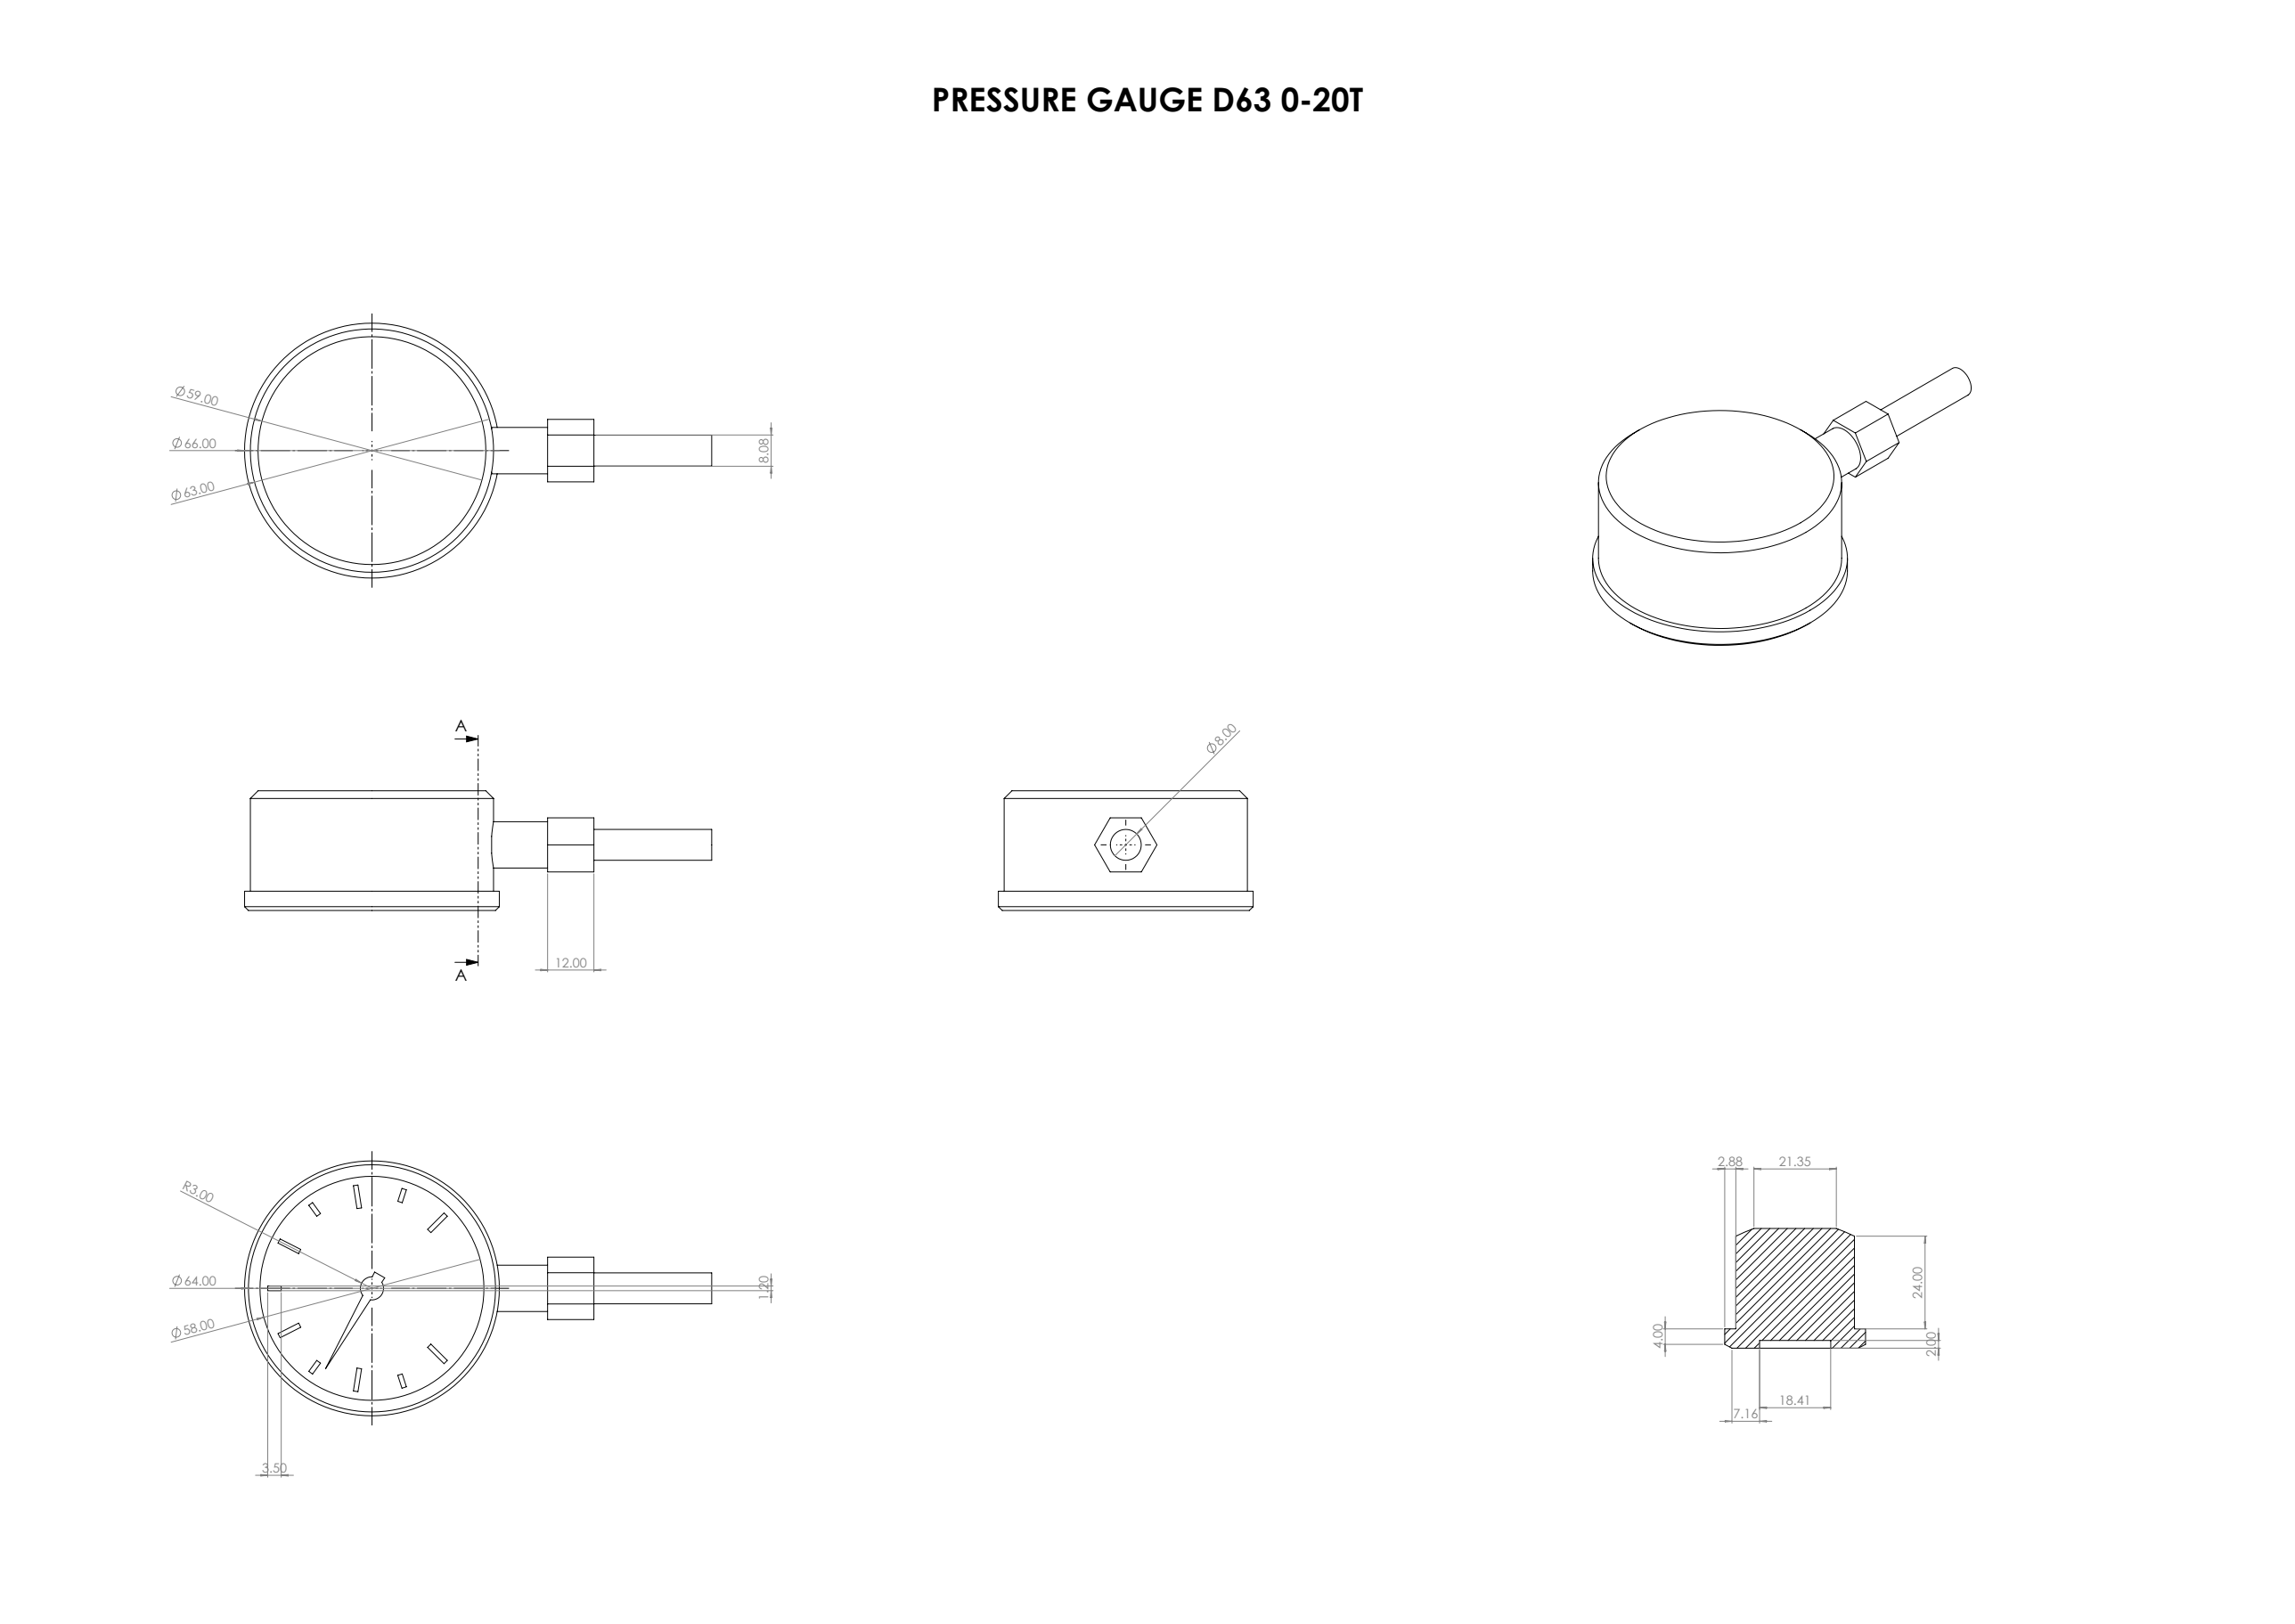
ISO-10303-21;
HEADER;
/* Generated by software containing ST-Developer
 * from STEP Tools, Inc. (www.steptools.com) 
 */

FILE_DESCRIPTION(
/* description */ (''),
/* implementation_level */ '2;1');

FILE_NAME(
/* name */ '13_Pressure_Gauge_D63_0-20T.step',
/* time_stamp */ '2026-10-20T10:03:03-07:00',
/* author */ (''),
/* organization */ (''),
/* preprocessor_version */ 'ST-DEVELOPER v20.2',
/* originating_system */ 'Autodesk Translation Framework v15.15.0.0',
/* authorisation */ '');

FILE_SCHEMA (('AUTOMOTIVE_DESIGN { 1 0 10303 214 3 1 1 }'));
ENDSEC;

DATA;
#10=MECHANICAL_DESIGN_GEOMETRIC_PRESENTATION_REPRESENTATION('',(#531,#532),#71492);
#389=SHAPE_REPRESENTATION_RELATIONSHIP('SRR','None',#71610,#408);
#408=ADVANCED_BREP_SHAPE_REPRESENTATION('',(#427),#71480);
#427=MANIFOLD_SOLID_BREP('Gauge',#28466);
#531=STYLED_ITEM('',(#71901),#27845);
#532=STYLED_ITEM('',(#71901),#427);
#878=B_SPLINE_CURVE_WITH_KNOTS('',3,(#48749,#48750,#48751,#48752,#48753,
#48754,#48755,#48756,#48757,#48758,#48759,#48760,#48761,#48762,#48763,#48764,
#48765,#48766),.UNSPECIFIED.,.F.,.F.,(4,2,2,2,2,2,2,2,4),(0.214479017187888,
0.226613658149299,0.453227316298599,0.679830564793567,0.906433813288534,
1.1330370617835,1.35964031027847,1.58625396842777,1.59838860938918),
 .UNSPECIFIED.);
#879=B_SPLINE_CURVE_WITH_KNOTS('',3,(#48768,#48769,#48770,#48771,#48772,
#48773,#48774,#48775,#48776,#48777,#48778,#48779,#48780,#48781,#48782,#48783,
#48784,#48785),.UNSPECIFIED.,.F.,.F.,(4,2,2,2,2,2,2,2,4),(2.02734664376496,
2.03948128472637,2.26609494287567,2.49269819137064,2.7193014398656,2.94590468836057,
3.17250793685554,3.39912159500484,3.41125623596625),.UNSPECIFIED.);
#1661=CYLINDRICAL_SURFACE('',#29879,0.4);
#1662=CYLINDRICAL_SURFACE('',#29897,0.6);
#1663=CYLINDRICAL_SURFACE('',#29898,0.300000000000001);
#1664=CYLINDRICAL_SURFACE('',#29904,0.300000000000001);
#1665=CYLINDRICAL_SURFACE('',#29967,2.9);
#1666=CYLINDRICAL_SURFACE('',#29973,3.15);
#1667=CYLINDRICAL_SURFACE('',#29977,3.3);
#1931=FACE_BOUND('',#5501,.T.);
#1932=FACE_BOUND('',#5509,.T.);
#1933=FACE_BOUND('',#5577,.T.);
#1934=FACE_BOUND('',#5578,.T.);
#1935=FACE_BOUND('',#5579,.T.);
#1936=FACE_BOUND('',#5580,.T.);
#1937=FACE_BOUND('',#5581,.T.);
#1938=FACE_BOUND('',#5582,.T.);
#1939=FACE_BOUND('',#5583,.T.);
#1940=FACE_BOUND('',#5584,.T.);
#1941=FACE_BOUND('',#5585,.T.);
#1942=FACE_BOUND('',#5586,.T.);
#1943=FACE_BOUND('',#5587,.T.);
#1944=FACE_BOUND('',#5588,.T.);
#1945=FACE_BOUND('',#5593,.T.);
#1946=FACE_BOUND('',#5595,.T.);
#1947=FACE_BOUND('',#5599,.T.);
#2447=CIRCLE('',#29880,0.4);
#2448=CIRCLE('',#29881,0.4);
#2449=CIRCLE('',#29884,0.6);
#2450=CIRCLE('',#29893,0.6);
#2451=CIRCLE('',#29895,0.6);
#2452=CIRCLE('',#29896,0.6);
#2453=CIRCLE('',#29899,0.300000000000001);
#2454=CIRCLE('',#29900,0.300000000000001);
#2455=CIRCLE('',#29905,0.300000000000001);
#2456=CIRCLE('',#29906,0.300000000000001);
#2457=CIRCLE('',#29966,2.9);
#2458=CIRCLE('',#29968,2.9);
#2459=CIRCLE('',#29970,2.95);
#2460=CIRCLE('',#29972,3.15);
#2461=CIRCLE('',#29974,3.15);
#2462=CIRCLE('',#29976,3.3);
#2463=CIRCLE('',#29978,3.3);
#2464=CIRCLE('',#29980,3.2);
#2859=CONICAL_SURFACE('',#29971,3.05,0.785398163397449);
#2860=CONICAL_SURFACE('',#29979,3.25,0.785398163397447);
#3861=FACE_OUTER_BOUND('',#5498,.T.);
#3862=FACE_OUTER_BOUND('',#5499,.T.);
#3863=FACE_OUTER_BOUND('',#5500,.T.);
#3864=FACE_OUTER_BOUND('',#5502,.T.);
#3865=FACE_OUTER_BOUND('',#5503,.T.);
#3866=FACE_OUTER_BOUND('',#5504,.T.);
#3867=FACE_OUTER_BOUND('',#5505,.T.);
#3868=FACE_OUTER_BOUND('',#5506,.T.);
#3869=FACE_OUTER_BOUND('',#5507,.T.);
#3870=FACE_OUTER_BOUND('',#5508,.T.);
#3871=FACE_OUTER_BOUND('',#5510,.T.);
#3872=FACE_OUTER_BOUND('',#5511,.T.);
#3873=FACE_OUTER_BOUND('',#5512,.T.);
#3874=FACE_OUTER_BOUND('',#5513,.T.);
#3875=FACE_OUTER_BOUND('',#5514,.T.);
#3876=FACE_OUTER_BOUND('',#5515,.T.);
#3877=FACE_OUTER_BOUND('',#5516,.T.);
#3878=FACE_OUTER_BOUND('',#5517,.T.);
#3879=FACE_OUTER_BOUND('',#5518,.T.);
#3880=FACE_OUTER_BOUND('',#5519,.T.);
#3881=FACE_OUTER_BOUND('',#5520,.T.);
#3882=FACE_OUTER_BOUND('',#5521,.T.);
#3883=FACE_OUTER_BOUND('',#5522,.T.);
#3884=FACE_OUTER_BOUND('',#5523,.T.);
#3885=FACE_OUTER_BOUND('',#5524,.T.);
#3886=FACE_OUTER_BOUND('',#5525,.T.);
#3887=FACE_OUTER_BOUND('',#5526,.T.);
#3888=FACE_OUTER_BOUND('',#5527,.T.);
#3889=FACE_OUTER_BOUND('',#5528,.T.);
#3890=FACE_OUTER_BOUND('',#5529,.T.);
#3891=FACE_OUTER_BOUND('',#5530,.T.);
#3892=FACE_OUTER_BOUND('',#5531,.T.);
#3893=FACE_OUTER_BOUND('',#5532,.T.);
#3894=FACE_OUTER_BOUND('',#5533,.T.);
#3895=FACE_OUTER_BOUND('',#5534,.T.);
#3896=FACE_OUTER_BOUND('',#5535,.T.);
#3897=FACE_OUTER_BOUND('',#5536,.T.);
#3898=FACE_OUTER_BOUND('',#5537,.T.);
#3899=FACE_OUTER_BOUND('',#5538,.T.);
#3900=FACE_OUTER_BOUND('',#5539,.T.);
#3901=FACE_OUTER_BOUND('',#5540,.T.);
#3902=FACE_OUTER_BOUND('',#5541,.T.);
#3903=FACE_OUTER_BOUND('',#5542,.T.);
#3904=FACE_OUTER_BOUND('',#5543,.T.);
#3905=FACE_OUTER_BOUND('',#5544,.T.);
#3906=FACE_OUTER_BOUND('',#5545,.T.);
#3907=FACE_OUTER_BOUND('',#5546,.T.);
#3908=FACE_OUTER_BOUND('',#5547,.T.);
#3909=FACE_OUTER_BOUND('',#5548,.T.);
#3910=FACE_OUTER_BOUND('',#5549,.T.);
#3911=FACE_OUTER_BOUND('',#5550,.T.);
#3912=FACE_OUTER_BOUND('',#5551,.T.);
#3913=FACE_OUTER_BOUND('',#5552,.T.);
#3914=FACE_OUTER_BOUND('',#5553,.T.);
#3915=FACE_OUTER_BOUND('',#5554,.T.);
#3916=FACE_OUTER_BOUND('',#5555,.T.);
#3917=FACE_OUTER_BOUND('',#5556,.T.);
#3918=FACE_OUTER_BOUND('',#5557,.T.);
#3919=FACE_OUTER_BOUND('',#5558,.T.);
#3920=FACE_OUTER_BOUND('',#5559,.T.);
#3921=FACE_OUTER_BOUND('',#5560,.T.);
#3922=FACE_OUTER_BOUND('',#5561,.T.);
#3923=FACE_OUTER_BOUND('',#5562,.T.);
#3924=FACE_OUTER_BOUND('',#5563,.T.);
#3925=FACE_OUTER_BOUND('',#5564,.T.);
#3926=FACE_OUTER_BOUND('',#5565,.T.);
#3927=FACE_OUTER_BOUND('',#5566,.T.);
#3928=FACE_OUTER_BOUND('',#5567,.T.);
#3929=FACE_OUTER_BOUND('',#5568,.T.);
#3930=FACE_OUTER_BOUND('',#5569,.T.);
#3931=FACE_OUTER_BOUND('',#5570,.T.);
#3932=FACE_OUTER_BOUND('',#5571,.T.);
#3933=FACE_OUTER_BOUND('',#5572,.T.);
#3934=FACE_OUTER_BOUND('',#5573,.T.);
#3935=FACE_OUTER_BOUND('',#5574,.T.);
#3936=FACE_OUTER_BOUND('',#5575,.T.);
#3937=FACE_OUTER_BOUND('',#5576,.T.);
#3938=FACE_OUTER_BOUND('',#5589,.T.);
#3939=FACE_OUTER_BOUND('',#5590,.T.);
#3940=FACE_OUTER_BOUND('',#5591,.T.);
#3941=FACE_OUTER_BOUND('',#5592,.T.);
#3942=FACE_OUTER_BOUND('',#5594,.T.);
#3943=FACE_OUTER_BOUND('',#5596,.T.);
#3944=FACE_OUTER_BOUND('',#5597,.T.);
#3945=FACE_OUTER_BOUND('',#5598,.T.);
#5498=EDGE_LOOP('',(#22583,#22584,#22585,#22586));
#5499=EDGE_LOOP('',(#22587));
#5500=EDGE_LOOP('',(#22588,#22589,#22590,#22591,#22592,#22593));
#5501=EDGE_LOOP('',(#22594));
#5502=EDGE_LOOP('',(#22595,#22596,#22597,#22598));
#5503=EDGE_LOOP('',(#22599,#22600,#22601,#22602));
#5504=EDGE_LOOP('',(#22603,#22604,#22605,#22606));
#5505=EDGE_LOOP('',(#22607,#22608,#22609,#22610));
#5506=EDGE_LOOP('',(#22611,#22612,#22613,#22614));
#5507=EDGE_LOOP('',(#22615,#22616,#22617,#22618));
#5508=EDGE_LOOP('',(#22619,#22620,#22621,#22622,#22623,#22624));
#5509=EDGE_LOOP('',(#22625));
#5510=EDGE_LOOP('',(#22626,#22627));
#5511=EDGE_LOOP('',(#22628,#22629,#22630));
#5512=EDGE_LOOP('',(#22631,#22632,#22633,#22634,#22635,#22636,#22637,#22638));
#5513=EDGE_LOOP('',(#22639,#22640,#22641,#22642));
#5514=EDGE_LOOP('',(#22643,#22644,#22645,#22646));
#5515=EDGE_LOOP('',(#22647,#22648,#22649,#22650));
#5516=EDGE_LOOP('',(#22651,#22652,#22653,#22654));
#5517=EDGE_LOOP('',(#22655,#22656,#22657,#22658));
#5518=EDGE_LOOP('',(#22659,#22660,#22661,#22662));
#5519=EDGE_LOOP('',(#22663,#22664,#22665,#22666));
#5520=EDGE_LOOP('',(#22667,#22668,#22669,#22670,#22671,#22672,#22673));
#5521=EDGE_LOOP('',(#22674,#22675,#22676,#22677));
#5522=EDGE_LOOP('',(#22678,#22679,#22680,#22681));
#5523=EDGE_LOOP('',(#22682,#22683,#22684,#22685));
#5524=EDGE_LOOP('',(#22686,#22687,#22688,#22689));
#5525=EDGE_LOOP('',(#22690,#22691,#22692,#22693));
#5526=EDGE_LOOP('',(#22694,#22695,#22696,#22697));
#5527=EDGE_LOOP('',(#22698,#22699,#22700,#22701));
#5528=EDGE_LOOP('',(#22702,#22703,#22704,#22705));
#5529=EDGE_LOOP('',(#22706,#22707,#22708,#22709));
#5530=EDGE_LOOP('',(#22710,#22711,#22712,#22713));
#5531=EDGE_LOOP('',(#22714,#22715,#22716,#22717));
#5532=EDGE_LOOP('',(#22718,#22719,#22720,#22721));
#5533=EDGE_LOOP('',(#22722,#22723,#22724,#22725));
#5534=EDGE_LOOP('',(#22726,#22727,#22728,#22729));
#5535=EDGE_LOOP('',(#22730,#22731,#22732,#22733));
#5536=EDGE_LOOP('',(#22734,#22735,#22736,#22737));
#5537=EDGE_LOOP('',(#22738,#22739,#22740,#22741));
#5538=EDGE_LOOP('',(#22742,#22743,#22744,#22745));
#5539=EDGE_LOOP('',(#22746,#22747,#22748,#22749));
#5540=EDGE_LOOP('',(#22750,#22751,#22752,#22753));
#5541=EDGE_LOOP('',(#22754,#22755,#22756,#22757));
#5542=EDGE_LOOP('',(#22758,#22759,#22760,#22761));
#5543=EDGE_LOOP('',(#22762,#22763,#22764,#22765));
#5544=EDGE_LOOP('',(#22766,#22767,#22768,#22769));
#5545=EDGE_LOOP('',(#22770,#22771,#22772,#22773));
#5546=EDGE_LOOP('',(#22774,#22775,#22776,#22777));
#5547=EDGE_LOOP('',(#22778,#22779,#22780,#22781));
#5548=EDGE_LOOP('',(#22782,#22783,#22784,#22785));
#5549=EDGE_LOOP('',(#22786,#22787,#22788,#22789));
#5550=EDGE_LOOP('',(#22790,#22791,#22792,#22793));
#5551=EDGE_LOOP('',(#22794,#22795,#22796,#22797));
#5552=EDGE_LOOP('',(#22798,#22799,#22800,#22801));
#5553=EDGE_LOOP('',(#22802,#22803,#22804,#22805));
#5554=EDGE_LOOP('',(#22806,#22807,#22808,#22809));
#5555=EDGE_LOOP('',(#22810,#22811,#22812,#22813));
#5556=EDGE_LOOP('',(#22814,#22815,#22816,#22817));
#5557=EDGE_LOOP('',(#22818,#22819,#22820,#22821));
#5558=EDGE_LOOP('',(#22822,#22823,#22824,#22825));
#5559=EDGE_LOOP('',(#22826,#22827,#22828,#22829));
#5560=EDGE_LOOP('',(#22830,#22831,#22832,#22833));
#5561=EDGE_LOOP('',(#22834,#22835,#22836,#22837));
#5562=EDGE_LOOP('',(#22838,#22839,#22840,#22841));
#5563=EDGE_LOOP('',(#22842,#22843,#22844,#22845));
#5564=EDGE_LOOP('',(#22846,#22847,#22848,#22849));
#5565=EDGE_LOOP('',(#22850,#22851,#22852,#22853));
#5566=EDGE_LOOP('',(#22854,#22855,#22856,#22857));
#5567=EDGE_LOOP('',(#22858,#22859,#22860,#22861));
#5568=EDGE_LOOP('',(#22862,#22863,#22864,#22865));
#5569=EDGE_LOOP('',(#22866,#22867,#22868,#22869));
#5570=EDGE_LOOP('',(#22870,#22871,#22872,#22873));
#5571=EDGE_LOOP('',(#22874,#22875,#22876,#22877));
#5572=EDGE_LOOP('',(#22878,#22879,#22880,#22881));
#5573=EDGE_LOOP('',(#22882,#22883,#22884,#22885));
#5574=EDGE_LOOP('',(#22886,#22887,#22888,#22889));
#5575=EDGE_LOOP('',(#22890,#22891,#22892,#22893));
#5576=EDGE_LOOP('',(#22894));
#5577=EDGE_LOOP('',(#22895,#22896,#22897,#22898));
#5578=EDGE_LOOP('',(#22899,#22900,#22901,#22902));
#5579=EDGE_LOOP('',(#22903,#22904,#22905,#22906));
#5580=EDGE_LOOP('',(#22907,#22908,#22909,#22910));
#5581=EDGE_LOOP('',(#22911,#22912,#22913,#22914));
#5582=EDGE_LOOP('',(#22915,#22916,#22917,#22918));
#5583=EDGE_LOOP('',(#22919,#22920,#22921,#22922));
#5584=EDGE_LOOP('',(#22923,#22924,#22925,#22926));
#5585=EDGE_LOOP('',(#22927,#22928,#22929,#22930));
#5586=EDGE_LOOP('',(#22931,#22932,#22933,#22934));
#5587=EDGE_LOOP('',(#22935,#22936,#22937,#22938));
#5588=EDGE_LOOP('',(#22939,#22940,#22941,#22942,#22943,#22944,#22945));
#5589=EDGE_LOOP('',(#22946,#22947,#22948,#22949));
#5590=EDGE_LOOP('',(#22950));
#5591=EDGE_LOOP('',(#22951,#22952,#22953,#22954));
#5592=EDGE_LOOP('',(#22955,#22956,#22957,#22958));
#5593=EDGE_LOOP('',(#22959,#22960,#22961,#22962));
#5594=EDGE_LOOP('',(#22963));
#5595=EDGE_LOOP('',(#22964));
#5596=EDGE_LOOP('',(#22965,#22966,#22967,#22968));
#5597=EDGE_LOOP('',(#22969,#22970,#22971,#22972));
#5598=EDGE_LOOP('',(#22973));
#5599=EDGE_LOOP('',(#22974));
#7821=LINE('',#48693,#10309);
#7822=LINE('',#48699,#10310);
#7823=LINE('',#48701,#10311);
#7824=LINE('',#48703,#10312);
#7825=LINE('',#48705,#10313);
#7826=LINE('',#48707,#10314);
#7827=LINE('',#48708,#10315);
#7828=LINE('',#48714,#10316);
#7829=LINE('',#48715,#10317);
#7830=LINE('',#48716,#10318);
#7831=LINE('',#48719,#10319);
#7832=LINE('',#48720,#10320);
#7833=LINE('',#48723,#10321);
#7834=LINE('',#48724,#10322);
#7835=LINE('',#48727,#10323);
#7836=LINE('',#48728,#10324);
#7837=LINE('',#48731,#10325);
#7838=LINE('',#48732,#10326);
#7839=LINE('',#48734,#10327);
#7840=LINE('',#48739,#10328);
#7841=LINE('',#48744,#10329);
#7842=LINE('',#48767,#10330);
#7843=LINE('',#48791,#10331);
#7844=LINE('',#48794,#10332);
#7845=LINE('',#48797,#10333);
#7846=LINE('',#48799,#10334);
#7847=LINE('',#48800,#10335);
#7848=LINE('',#48803,#10336);
#7849=LINE('',#48805,#10337);
#7850=LINE('',#48806,#10338);
#7851=LINE('',#48809,#10339);
#7852=LINE('',#48811,#10340);
#7853=LINE('',#48812,#10341);
#7854=LINE('',#48818,#10342);
#7855=LINE('',#48821,#10343);
#7856=LINE('',#48823,#10344);
#7857=LINE('',#48824,#10345);
#7858=LINE('',#48826,#10346);
#7859=LINE('',#48827,#10347);
#7860=LINE('',#48832,#10348);
#7861=LINE('',#48834,#10349);
#7862=LINE('',#48836,#10350);
#7863=LINE('',#48837,#10351);
#7864=LINE('',#48840,#10352);
#7865=LINE('',#48842,#10353);
#7866=LINE('',#48843,#10354);
#7867=LINE('',#48846,#10355);
#7868=LINE('',#48848,#10356);
#7869=LINE('',#48849,#10357);
#7870=LINE('',#48851,#10358);
#7871=LINE('',#48852,#10359);
#7872=LINE('',#48857,#10360);
#7873=LINE('',#48859,#10361);
#7874=LINE('',#48861,#10362);
#7875=LINE('',#48862,#10363);
#7876=LINE('',#48865,#10364);
#7877=LINE('',#48867,#10365);
#7878=LINE('',#48868,#10366);
#7879=LINE('',#48871,#10367);
#7880=LINE('',#48873,#10368);
#7881=LINE('',#48874,#10369);
#7882=LINE('',#48876,#10370);
#7883=LINE('',#48877,#10371);
#7884=LINE('',#48882,#10372);
#7885=LINE('',#48884,#10373);
#7886=LINE('',#48886,#10374);
#7887=LINE('',#48887,#10375);
#7888=LINE('',#48890,#10376);
#7889=LINE('',#48892,#10377);
#7890=LINE('',#48893,#10378);
#7891=LINE('',#48896,#10379);
#7892=LINE('',#48898,#10380);
#7893=LINE('',#48899,#10381);
#7894=LINE('',#48901,#10382);
#7895=LINE('',#48902,#10383);
#7896=LINE('',#48907,#10384);
#7897=LINE('',#48909,#10385);
#7898=LINE('',#48911,#10386);
#7899=LINE('',#48912,#10387);
#7900=LINE('',#48915,#10388);
#7901=LINE('',#48917,#10389);
#7902=LINE('',#48918,#10390);
#7903=LINE('',#48921,#10391);
#7904=LINE('',#48923,#10392);
#7905=LINE('',#48924,#10393);
#7906=LINE('',#48926,#10394);
#7907=LINE('',#48927,#10395);
#7908=LINE('',#48932,#10396);
#7909=LINE('',#48934,#10397);
#7910=LINE('',#48936,#10398);
#7911=LINE('',#48937,#10399);
#7912=LINE('',#48940,#10400);
#7913=LINE('',#48942,#10401);
#7914=LINE('',#48943,#10402);
#7915=LINE('',#48946,#10403);
#7916=LINE('',#48948,#10404);
#7917=LINE('',#48949,#10405);
#7918=LINE('',#48951,#10406);
#7919=LINE('',#48952,#10407);
#7920=LINE('',#48957,#10408);
#7921=LINE('',#48959,#10409);
#7922=LINE('',#48961,#10410);
#7923=LINE('',#48962,#10411);
#7924=LINE('',#48965,#10412);
#7925=LINE('',#48967,#10413);
#7926=LINE('',#48968,#10414);
#7927=LINE('',#48971,#10415);
#7928=LINE('',#48973,#10416);
#7929=LINE('',#48974,#10417);
#7930=LINE('',#48976,#10418);
#7931=LINE('',#48977,#10419);
#7932=LINE('',#48982,#10420);
#7933=LINE('',#48984,#10421);
#7934=LINE('',#48986,#10422);
#7935=LINE('',#48987,#10423);
#7936=LINE('',#48990,#10424);
#7937=LINE('',#48992,#10425);
#7938=LINE('',#48993,#10426);
#7939=LINE('',#48996,#10427);
#7940=LINE('',#48998,#10428);
#7941=LINE('',#48999,#10429);
#7942=LINE('',#49001,#10430);
#7943=LINE('',#49002,#10431);
#7944=LINE('',#49007,#10432);
#7945=LINE('',#49009,#10433);
#7946=LINE('',#49011,#10434);
#7947=LINE('',#49012,#10435);
#7948=LINE('',#49015,#10436);
#7949=LINE('',#49017,#10437);
#7950=LINE('',#49018,#10438);
#7951=LINE('',#49021,#10439);
#7952=LINE('',#49023,#10440);
#7953=LINE('',#49024,#10441);
#7954=LINE('',#49026,#10442);
#7955=LINE('',#49027,#10443);
#7956=LINE('',#49032,#10444);
#7957=LINE('',#49034,#10445);
#7958=LINE('',#49036,#10446);
#7959=LINE('',#49037,#10447);
#7960=LINE('',#49040,#10448);
#7961=LINE('',#49042,#10449);
#7962=LINE('',#49043,#10450);
#7963=LINE('',#49046,#10451);
#7964=LINE('',#49048,#10452);
#7965=LINE('',#49049,#10453);
#7966=LINE('',#49051,#10454);
#7967=LINE('',#49052,#10455);
#7968=LINE('',#49057,#10456);
#7969=LINE('',#49059,#10457);
#7970=LINE('',#49061,#10458);
#7971=LINE('',#49062,#10459);
#7972=LINE('',#49065,#10460);
#7973=LINE('',#49067,#10461);
#7974=LINE('',#49068,#10462);
#7975=LINE('',#49071,#10463);
#7976=LINE('',#49073,#10464);
#7977=LINE('',#49074,#10465);
#7978=LINE('',#49076,#10466);
#7979=LINE('',#49077,#10467);
#7980=LINE('',#49082,#10468);
#7981=LINE('',#49084,#10469);
#7982=LINE('',#49086,#10470);
#7983=LINE('',#49087,#10471);
#7984=LINE('',#49090,#10472);
#7985=LINE('',#49092,#10473);
#7986=LINE('',#49093,#10474);
#7987=LINE('',#49096,#10475);
#7988=LINE('',#49098,#10476);
#7989=LINE('',#49099,#10477);
#7990=LINE('',#49101,#10478);
#7991=LINE('',#49102,#10479);
#7992=LINE('',#49109,#10480);
#7993=LINE('',#49117,#10481);
#7994=LINE('',#49121,#10482);
#7995=LINE('',#49128,#10483);
#7996=LINE('',#49132,#10484);
#10309=VECTOR('',#34760,0.4);
#10310=VECTOR('',#34767,1.);
#10311=VECTOR('',#34768,1.);
#10312=VECTOR('',#34769,1.);
#10313=VECTOR('',#34770,1.);
#10314=VECTOR('',#34771,1.);
#10315=VECTOR('',#34772,1.);
#10316=VECTOR('',#34777,1.);
#10317=VECTOR('',#34778,1.);
#10318=VECTOR('',#34779,1.);
#10319=VECTOR('',#34782,1.);
#10320=VECTOR('',#34783,1.);
#10321=VECTOR('',#34786,1.);
#10322=VECTOR('',#34787,1.);
#10323=VECTOR('',#34790,1.);
#10324=VECTOR('',#34791,1.);
#10325=VECTOR('',#34794,1.);
#10326=VECTOR('',#34795,1.);
#10327=VECTOR('',#34798,1.);
#10328=VECTOR('',#34803,1.);
#10329=VECTOR('',#34808,1.);
#10330=VECTOR('',#34815,0.6);
#10331=VECTOR('',#34820,1.);
#10332=VECTOR('',#34823,1.);
#10333=VECTOR('',#34826,1.);
#10334=VECTOR('',#34827,1.);
#10335=VECTOR('',#34828,1.);
#10336=VECTOR('',#34831,1.);
#10337=VECTOR('',#34832,1.);
#10338=VECTOR('',#34833,1.);
#10339=VECTOR('',#34836,1.);
#10340=VECTOR('',#34837,1.);
#10341=VECTOR('',#34838,1.);
#10342=VECTOR('',#34845,1.);
#10343=VECTOR('',#34848,1.);
#10344=VECTOR('',#34849,1.);
#10345=VECTOR('',#34850,1.);
#10346=VECTOR('',#34853,1.);
#10347=VECTOR('',#34854,1.);
#10348=VECTOR('',#34859,1.);
#10349=VECTOR('',#34860,1.);
#10350=VECTOR('',#34861,1.);
#10351=VECTOR('',#34862,1.);
#10352=VECTOR('',#34865,1.);
#10353=VECTOR('',#34866,1.);
#10354=VECTOR('',#34867,1.);
#10355=VECTOR('',#34870,1.);
#10356=VECTOR('',#34871,1.);
#10357=VECTOR('',#34872,1.);
#10358=VECTOR('',#34875,1.);
#10359=VECTOR('',#34876,1.);
#10360=VECTOR('',#34881,1.);
#10361=VECTOR('',#34882,1.);
#10362=VECTOR('',#34883,1.);
#10363=VECTOR('',#34884,1.);
#10364=VECTOR('',#34887,1.);
#10365=VECTOR('',#34888,1.);
#10366=VECTOR('',#34889,1.);
#10367=VECTOR('',#34892,1.);
#10368=VECTOR('',#34893,1.);
#10369=VECTOR('',#34894,1.);
#10370=VECTOR('',#34897,1.);
#10371=VECTOR('',#34898,1.);
#10372=VECTOR('',#34903,1.);
#10373=VECTOR('',#34904,1.);
#10374=VECTOR('',#34905,1.);
#10375=VECTOR('',#34906,1.);
#10376=VECTOR('',#34909,1.);
#10377=VECTOR('',#34910,1.);
#10378=VECTOR('',#34911,1.);
#10379=VECTOR('',#34914,1.);
#10380=VECTOR('',#34915,1.);
#10381=VECTOR('',#34916,1.);
#10382=VECTOR('',#34919,1.);
#10383=VECTOR('',#34920,1.);
#10384=VECTOR('',#34925,1.);
#10385=VECTOR('',#34926,1.);
#10386=VECTOR('',#34927,1.);
#10387=VECTOR('',#34928,1.);
#10388=VECTOR('',#34931,1.);
#10389=VECTOR('',#34932,1.);
#10390=VECTOR('',#34933,1.);
#10391=VECTOR('',#34936,1.);
#10392=VECTOR('',#34937,1.);
#10393=VECTOR('',#34938,1.);
#10394=VECTOR('',#34941,1.);
#10395=VECTOR('',#34942,1.);
#10396=VECTOR('',#34947,1.);
#10397=VECTOR('',#34948,1.);
#10398=VECTOR('',#34949,1.);
#10399=VECTOR('',#34950,1.);
#10400=VECTOR('',#34953,1.);
#10401=VECTOR('',#34954,1.);
#10402=VECTOR('',#34955,1.);
#10403=VECTOR('',#34958,1.);
#10404=VECTOR('',#34959,1.);
#10405=VECTOR('',#34960,1.);
#10406=VECTOR('',#34963,1.);
#10407=VECTOR('',#34964,1.);
#10408=VECTOR('',#34969,1.);
#10409=VECTOR('',#34970,1.);
#10410=VECTOR('',#34971,1.);
#10411=VECTOR('',#34972,1.);
#10412=VECTOR('',#34975,1.);
#10413=VECTOR('',#34976,1.);
#10414=VECTOR('',#34977,1.);
#10415=VECTOR('',#34980,1.);
#10416=VECTOR('',#34981,1.);
#10417=VECTOR('',#34982,1.);
#10418=VECTOR('',#34985,1.);
#10419=VECTOR('',#34986,1.);
#10420=VECTOR('',#34991,1.);
#10421=VECTOR('',#34992,1.);
#10422=VECTOR('',#34993,1.);
#10423=VECTOR('',#34994,1.);
#10424=VECTOR('',#34997,1.);
#10425=VECTOR('',#34998,1.);
#10426=VECTOR('',#34999,1.);
#10427=VECTOR('',#35002,1.);
#10428=VECTOR('',#35003,1.);
#10429=VECTOR('',#35004,1.);
#10430=VECTOR('',#35007,1.);
#10431=VECTOR('',#35008,1.);
#10432=VECTOR('',#35013,1.);
#10433=VECTOR('',#35014,1.);
#10434=VECTOR('',#35015,1.);
#10435=VECTOR('',#35016,1.);
#10436=VECTOR('',#35019,1.);
#10437=VECTOR('',#35020,1.);
#10438=VECTOR('',#35021,1.);
#10439=VECTOR('',#35024,1.);
#10440=VECTOR('',#35025,1.);
#10441=VECTOR('',#35026,1.);
#10442=VECTOR('',#35029,1.);
#10443=VECTOR('',#35030,1.);
#10444=VECTOR('',#35035,1.);
#10445=VECTOR('',#35036,1.);
#10446=VECTOR('',#35037,1.);
#10447=VECTOR('',#35038,1.);
#10448=VECTOR('',#35041,1.);
#10449=VECTOR('',#35042,1.);
#10450=VECTOR('',#35043,1.);
#10451=VECTOR('',#35046,1.);
#10452=VECTOR('',#35047,1.);
#10453=VECTOR('',#35048,1.);
#10454=VECTOR('',#35051,1.);
#10455=VECTOR('',#35052,1.);
#10456=VECTOR('',#35057,1.);
#10457=VECTOR('',#35058,1.);
#10458=VECTOR('',#35059,1.);
#10459=VECTOR('',#35060,1.);
#10460=VECTOR('',#35063,1.);
#10461=VECTOR('',#35064,1.);
#10462=VECTOR('',#35065,1.);
#10463=VECTOR('',#35068,1.);
#10464=VECTOR('',#35069,1.);
#10465=VECTOR('',#35070,1.);
#10466=VECTOR('',#35073,1.);
#10467=VECTOR('',#35074,1.);
#10468=VECTOR('',#35079,1.);
#10469=VECTOR('',#35080,1.);
#10470=VECTOR('',#35081,1.);
#10471=VECTOR('',#35082,1.);
#10472=VECTOR('',#35085,1.);
#10473=VECTOR('',#35086,1.);
#10474=VECTOR('',#35087,1.);
#10475=VECTOR('',#35090,1.);
#10476=VECTOR('',#35091,1.);
#10477=VECTOR('',#35092,1.);
#10478=VECTOR('',#35095,1.);
#10479=VECTOR('',#35096,1.);
#10480=VECTOR('',#35105,2.9);
#10481=VECTOR('',#35116,3.05);
#10482=VECTOR('',#35121,3.15);
#10483=VECTOR('',#35130,3.3);
#10484=VECTOR('',#35135,3.25);
#12733=VERTEX_POINT('',#48690);
#12734=VERTEX_POINT('',#48692);
#12735=VERTEX_POINT('',#48697);
#12736=VERTEX_POINT('',#48698);
#12737=VERTEX_POINT('',#48700);
#12738=VERTEX_POINT('',#48702);
#12739=VERTEX_POINT('',#48704);
#12740=VERTEX_POINT('',#48706);
#12741=VERTEX_POINT('',#48709);
#12742=VERTEX_POINT('',#48712);
#12743=VERTEX_POINT('',#48713);
#12744=VERTEX_POINT('',#48718);
#12745=VERTEX_POINT('',#48722);
#12746=VERTEX_POINT('',#48726);
#12747=VERTEX_POINT('',#48730);
#12748=VERTEX_POINT('',#48737);
#12749=VERTEX_POINT('',#48738);
#12750=VERTEX_POINT('',#48742);
#12751=VERTEX_POINT('',#48743);
#12752=VERTEX_POINT('',#48745);
#12753=VERTEX_POINT('',#48787);
#12754=VERTEX_POINT('',#48788);
#12755=VERTEX_POINT('',#48790);
#12756=VERTEX_POINT('',#48792);
#12757=VERTEX_POINT('',#48796);
#12758=VERTEX_POINT('',#48798);
#12759=VERTEX_POINT('',#48802);
#12760=VERTEX_POINT('',#48804);
#12761=VERTEX_POINT('',#48808);
#12762=VERTEX_POINT('',#48810);
#12763=VERTEX_POINT('',#48814);
#12764=VERTEX_POINT('',#48816);
#12765=VERTEX_POINT('',#48820);
#12766=VERTEX_POINT('',#48822);
#12767=VERTEX_POINT('',#48830);
#12768=VERTEX_POINT('',#48831);
#12769=VERTEX_POINT('',#48833);
#12770=VERTEX_POINT('',#48835);
#12771=VERTEX_POINT('',#48839);
#12772=VERTEX_POINT('',#48841);
#12773=VERTEX_POINT('',#48845);
#12774=VERTEX_POINT('',#48847);
#12775=VERTEX_POINT('',#48855);
#12776=VERTEX_POINT('',#48856);
#12777=VERTEX_POINT('',#48858);
#12778=VERTEX_POINT('',#48860);
#12779=VERTEX_POINT('',#48864);
#12780=VERTEX_POINT('',#48866);
#12781=VERTEX_POINT('',#48870);
#12782=VERTEX_POINT('',#48872);
#12783=VERTEX_POINT('',#48880);
#12784=VERTEX_POINT('',#48881);
#12785=VERTEX_POINT('',#48883);
#12786=VERTEX_POINT('',#48885);
#12787=VERTEX_POINT('',#48889);
#12788=VERTEX_POINT('',#48891);
#12789=VERTEX_POINT('',#48895);
#12790=VERTEX_POINT('',#48897);
#12791=VERTEX_POINT('',#48905);
#12792=VERTEX_POINT('',#48906);
#12793=VERTEX_POINT('',#48908);
#12794=VERTEX_POINT('',#48910);
#12795=VERTEX_POINT('',#48914);
#12796=VERTEX_POINT('',#48916);
#12797=VERTEX_POINT('',#48920);
#12798=VERTEX_POINT('',#48922);
#12799=VERTEX_POINT('',#48930);
#12800=VERTEX_POINT('',#48931);
#12801=VERTEX_POINT('',#48933);
#12802=VERTEX_POINT('',#48935);
#12803=VERTEX_POINT('',#48939);
#12804=VERTEX_POINT('',#48941);
#12805=VERTEX_POINT('',#48945);
#12806=VERTEX_POINT('',#48947);
#12807=VERTEX_POINT('',#48955);
#12808=VERTEX_POINT('',#48956);
#12809=VERTEX_POINT('',#48958);
#12810=VERTEX_POINT('',#48960);
#12811=VERTEX_POINT('',#48964);
#12812=VERTEX_POINT('',#48966);
#12813=VERTEX_POINT('',#48970);
#12814=VERTEX_POINT('',#48972);
#12815=VERTEX_POINT('',#48980);
#12816=VERTEX_POINT('',#48981);
#12817=VERTEX_POINT('',#48983);
#12818=VERTEX_POINT('',#48985);
#12819=VERTEX_POINT('',#48989);
#12820=VERTEX_POINT('',#48991);
#12821=VERTEX_POINT('',#48995);
#12822=VERTEX_POINT('',#48997);
#12823=VERTEX_POINT('',#49005);
#12824=VERTEX_POINT('',#49006);
#12825=VERTEX_POINT('',#49008);
#12826=VERTEX_POINT('',#49010);
#12827=VERTEX_POINT('',#49014);
#12828=VERTEX_POINT('',#49016);
#12829=VERTEX_POINT('',#49020);
#12830=VERTEX_POINT('',#49022);
#12831=VERTEX_POINT('',#49030);
#12832=VERTEX_POINT('',#49031);
#12833=VERTEX_POINT('',#49033);
#12834=VERTEX_POINT('',#49035);
#12835=VERTEX_POINT('',#49039);
#12836=VERTEX_POINT('',#49041);
#12837=VERTEX_POINT('',#49045);
#12838=VERTEX_POINT('',#49047);
#12839=VERTEX_POINT('',#49055);
#12840=VERTEX_POINT('',#49056);
#12841=VERTEX_POINT('',#49058);
#12842=VERTEX_POINT('',#49060);
#12843=VERTEX_POINT('',#49064);
#12844=VERTEX_POINT('',#49066);
#12845=VERTEX_POINT('',#49070);
#12846=VERTEX_POINT('',#49072);
#12847=VERTEX_POINT('',#49080);
#12848=VERTEX_POINT('',#49081);
#12849=VERTEX_POINT('',#49083);
#12850=VERTEX_POINT('',#49085);
#12851=VERTEX_POINT('',#49089);
#12852=VERTEX_POINT('',#49091);
#12853=VERTEX_POINT('',#49095);
#12854=VERTEX_POINT('',#49097);
#12855=VERTEX_POINT('',#49105);
#12856=VERTEX_POINT('',#49108);
#12857=VERTEX_POINT('',#49112);
#12858=VERTEX_POINT('',#49115);
#12859=VERTEX_POINT('',#49119);
#12860=VERTEX_POINT('',#49123);
#12861=VERTEX_POINT('',#49126);
#12862=VERTEX_POINT('',#49130);
#16175=EDGE_CURVE('',#12733,#12733,#2447,.T.);
#16176=EDGE_CURVE('',#12733,#12734,#7821,.T.);
#16177=EDGE_CURVE('',#12734,#12734,#2448,.T.);
#16178=EDGE_CURVE('',#12735,#12736,#7822,.T.);
#16179=EDGE_CURVE('',#12736,#12737,#7823,.T.);
#16180=EDGE_CURVE('',#12737,#12738,#7824,.T.);
#16181=EDGE_CURVE('',#12738,#12739,#7825,.T.);
#16182=EDGE_CURVE('',#12739,#12740,#7826,.T.);
#16183=EDGE_CURVE('',#12740,#12735,#7827,.T.);
#16184=EDGE_CURVE('',#12741,#12741,#2449,.T.);
#16185=EDGE_CURVE('',#12742,#12743,#7828,.T.);
#16186=EDGE_CURVE('',#12743,#12735,#7829,.T.);
#16187=EDGE_CURVE('',#12742,#12740,#7830,.T.);
#16188=EDGE_CURVE('',#12744,#12742,#7831,.T.);
#16189=EDGE_CURVE('',#12744,#12739,#7832,.T.);
#16190=EDGE_CURVE('',#12745,#12744,#7833,.T.);
#16191=EDGE_CURVE('',#12745,#12738,#7834,.T.);
#16192=EDGE_CURVE('',#12746,#12745,#7835,.T.);
#16193=EDGE_CURVE('',#12746,#12737,#7836,.T.);
#16194=EDGE_CURVE('',#12747,#12746,#7837,.T.);
#16195=EDGE_CURVE('',#12747,#12736,#7838,.T.);
#16196=EDGE_CURVE('',#12743,#12747,#7839,.T.);
#16197=EDGE_CURVE('',#12748,#12749,#7840,.T.);
#16198=EDGE_CURVE('',#12748,#12749,#2450,.T.);
#16199=EDGE_CURVE('',#12750,#12751,#7841,.T.);
#16200=EDGE_CURVE('',#12750,#12752,#2451,.T.);
#16201=EDGE_CURVE('',#12752,#12751,#2452,.T.);
#16202=EDGE_CURVE('',#12751,#12748,#878,.T.);
#16203=EDGE_CURVE('',#12752,#12741,#7842,.T.);
#16204=EDGE_CURVE('',#12749,#12750,#879,.T.);
#16205=EDGE_CURVE('',#12753,#12754,#2453,.T.);
#16206=EDGE_CURVE('',#12753,#12755,#7843,.T.);
#16207=EDGE_CURVE('',#12756,#12755,#2454,.T.);
#16208=EDGE_CURVE('',#12754,#12756,#7844,.T.);
#16209=EDGE_CURVE('',#12754,#12757,#7845,.T.);
#16210=EDGE_CURVE('',#12758,#12756,#7846,.T.);
#16211=EDGE_CURVE('',#12757,#12758,#7847,.T.);
#16212=EDGE_CURVE('',#12757,#12759,#7848,.T.);
#16213=EDGE_CURVE('',#12760,#12758,#7849,.T.);
#16214=EDGE_CURVE('',#12759,#12760,#7850,.T.);
#16215=EDGE_CURVE('',#12759,#12761,#7851,.T.);
#16216=EDGE_CURVE('',#12762,#12760,#7852,.T.);
#16217=EDGE_CURVE('',#12761,#12762,#7853,.T.);
#16218=EDGE_CURVE('',#12761,#12763,#2455,.T.);
#16219=EDGE_CURVE('',#12764,#12762,#2456,.T.);
#16220=EDGE_CURVE('',#12763,#12764,#7854,.T.);
#16221=EDGE_CURVE('',#12763,#12765,#7855,.T.);
#16222=EDGE_CURVE('',#12766,#12764,#7856,.T.);
#16223=EDGE_CURVE('',#12765,#12766,#7857,.T.);
#16224=EDGE_CURVE('',#12765,#12753,#7858,.T.);
#16225=EDGE_CURVE('',#12755,#12766,#7859,.T.);
#16226=EDGE_CURVE('',#12767,#12768,#7860,.T.);
#16227=EDGE_CURVE('',#12767,#12769,#7861,.T.);
#16228=EDGE_CURVE('',#12769,#12770,#7862,.T.);
#16229=EDGE_CURVE('',#12768,#12770,#7863,.T.);
#16230=EDGE_CURVE('',#12771,#12767,#7864,.T.);
#16231=EDGE_CURVE('',#12771,#12772,#7865,.T.);
#16232=EDGE_CURVE('',#12772,#12769,#7866,.T.);
#16233=EDGE_CURVE('',#12773,#12771,#7867,.T.);
#16234=EDGE_CURVE('',#12773,#12774,#7868,.T.);
#16235=EDGE_CURVE('',#12774,#12772,#7869,.T.);
#16236=EDGE_CURVE('',#12768,#12773,#7870,.T.);
#16237=EDGE_CURVE('',#12770,#12774,#7871,.T.);
#16238=EDGE_CURVE('',#12775,#12776,#7872,.T.);
#16239=EDGE_CURVE('',#12775,#12777,#7873,.T.);
#16240=EDGE_CURVE('',#12777,#12778,#7874,.T.);
#16241=EDGE_CURVE('',#12776,#12778,#7875,.T.);
#16242=EDGE_CURVE('',#12779,#12775,#7876,.T.);
#16243=EDGE_CURVE('',#12779,#12780,#7877,.T.);
#16244=EDGE_CURVE('',#12780,#12777,#7878,.T.);
#16245=EDGE_CURVE('',#12781,#12779,#7879,.T.);
#16246=EDGE_CURVE('',#12781,#12782,#7880,.T.);
#16247=EDGE_CURVE('',#12782,#12780,#7881,.T.);
#16248=EDGE_CURVE('',#12776,#12781,#7882,.T.);
#16249=EDGE_CURVE('',#12778,#12782,#7883,.T.);
#16250=EDGE_CURVE('',#12783,#12784,#7884,.T.);
#16251=EDGE_CURVE('',#12783,#12785,#7885,.T.);
#16252=EDGE_CURVE('',#12785,#12786,#7886,.T.);
#16253=EDGE_CURVE('',#12784,#12786,#7887,.T.);
#16254=EDGE_CURVE('',#12787,#12783,#7888,.T.);
#16255=EDGE_CURVE('',#12787,#12788,#7889,.T.);
#16256=EDGE_CURVE('',#12788,#12785,#7890,.T.);
#16257=EDGE_CURVE('',#12789,#12787,#7891,.T.);
#16258=EDGE_CURVE('',#12789,#12790,#7892,.T.);
#16259=EDGE_CURVE('',#12790,#12788,#7893,.T.);
#16260=EDGE_CURVE('',#12784,#12789,#7894,.T.);
#16261=EDGE_CURVE('',#12786,#12790,#7895,.T.);
#16262=EDGE_CURVE('',#12791,#12792,#7896,.T.);
#16263=EDGE_CURVE('',#12791,#12793,#7897,.T.);
#16264=EDGE_CURVE('',#12793,#12794,#7898,.T.);
#16265=EDGE_CURVE('',#12792,#12794,#7899,.T.);
#16266=EDGE_CURVE('',#12795,#12791,#7900,.T.);
#16267=EDGE_CURVE('',#12795,#12796,#7901,.T.);
#16268=EDGE_CURVE('',#12796,#12793,#7902,.T.);
#16269=EDGE_CURVE('',#12797,#12795,#7903,.T.);
#16270=EDGE_CURVE('',#12797,#12798,#7904,.T.);
#16271=EDGE_CURVE('',#12798,#12796,#7905,.T.);
#16272=EDGE_CURVE('',#12792,#12797,#7906,.T.);
#16273=EDGE_CURVE('',#12794,#12798,#7907,.T.);
#16274=EDGE_CURVE('',#12799,#12800,#7908,.T.);
#16275=EDGE_CURVE('',#12799,#12801,#7909,.T.);
#16276=EDGE_CURVE('',#12801,#12802,#7910,.T.);
#16277=EDGE_CURVE('',#12800,#12802,#7911,.T.);
#16278=EDGE_CURVE('',#12803,#12799,#7912,.T.);
#16279=EDGE_CURVE('',#12803,#12804,#7913,.T.);
#16280=EDGE_CURVE('',#12804,#12801,#7914,.T.);
#16281=EDGE_CURVE('',#12805,#12803,#7915,.T.);
#16282=EDGE_CURVE('',#12805,#12806,#7916,.T.);
#16283=EDGE_CURVE('',#12806,#12804,#7917,.T.);
#16284=EDGE_CURVE('',#12800,#12805,#7918,.T.);
#16285=EDGE_CURVE('',#12802,#12806,#7919,.T.);
#16286=EDGE_CURVE('',#12807,#12808,#7920,.T.);
#16287=EDGE_CURVE('',#12807,#12809,#7921,.T.);
#16288=EDGE_CURVE('',#12809,#12810,#7922,.T.);
#16289=EDGE_CURVE('',#12808,#12810,#7923,.T.);
#16290=EDGE_CURVE('',#12811,#12807,#7924,.T.);
#16291=EDGE_CURVE('',#12811,#12812,#7925,.T.);
#16292=EDGE_CURVE('',#12812,#12809,#7926,.T.);
#16293=EDGE_CURVE('',#12813,#12811,#7927,.T.);
#16294=EDGE_CURVE('',#12813,#12814,#7928,.T.);
#16295=EDGE_CURVE('',#12814,#12812,#7929,.T.);
#16296=EDGE_CURVE('',#12808,#12813,#7930,.T.);
#16297=EDGE_CURVE('',#12810,#12814,#7931,.T.);
#16298=EDGE_CURVE('',#12815,#12816,#7932,.T.);
#16299=EDGE_CURVE('',#12815,#12817,#7933,.T.);
#16300=EDGE_CURVE('',#12817,#12818,#7934,.T.);
#16301=EDGE_CURVE('',#12816,#12818,#7935,.T.);
#16302=EDGE_CURVE('',#12819,#12815,#7936,.T.);
#16303=EDGE_CURVE('',#12819,#12820,#7937,.T.);
#16304=EDGE_CURVE('',#12820,#12817,#7938,.T.);
#16305=EDGE_CURVE('',#12821,#12819,#7939,.T.);
#16306=EDGE_CURVE('',#12821,#12822,#7940,.T.);
#16307=EDGE_CURVE('',#12822,#12820,#7941,.T.);
#16308=EDGE_CURVE('',#12816,#12821,#7942,.T.);
#16309=EDGE_CURVE('',#12818,#12822,#7943,.T.);
#16310=EDGE_CURVE('',#12823,#12824,#7944,.T.);
#16311=EDGE_CURVE('',#12823,#12825,#7945,.T.);
#16312=EDGE_CURVE('',#12825,#12826,#7946,.T.);
#16313=EDGE_CURVE('',#12824,#12826,#7947,.T.);
#16314=EDGE_CURVE('',#12827,#12823,#7948,.T.);
#16315=EDGE_CURVE('',#12827,#12828,#7949,.T.);
#16316=EDGE_CURVE('',#12828,#12825,#7950,.T.);
#16317=EDGE_CURVE('',#12829,#12827,#7951,.T.);
#16318=EDGE_CURVE('',#12829,#12830,#7952,.T.);
#16319=EDGE_CURVE('',#12830,#12828,#7953,.T.);
#16320=EDGE_CURVE('',#12824,#12829,#7954,.T.);
#16321=EDGE_CURVE('',#12826,#12830,#7955,.T.);
#16322=EDGE_CURVE('',#12831,#12832,#7956,.T.);
#16323=EDGE_CURVE('',#12831,#12833,#7957,.T.);
#16324=EDGE_CURVE('',#12833,#12834,#7958,.T.);
#16325=EDGE_CURVE('',#12832,#12834,#7959,.T.);
#16326=EDGE_CURVE('',#12835,#12831,#7960,.T.);
#16327=EDGE_CURVE('',#12835,#12836,#7961,.T.);
#16328=EDGE_CURVE('',#12836,#12833,#7962,.T.);
#16329=EDGE_CURVE('',#12837,#12835,#7963,.T.);
#16330=EDGE_CURVE('',#12837,#12838,#7964,.T.);
#16331=EDGE_CURVE('',#12838,#12836,#7965,.T.);
#16332=EDGE_CURVE('',#12832,#12837,#7966,.T.);
#16333=EDGE_CURVE('',#12834,#12838,#7967,.T.);
#16334=EDGE_CURVE('',#12839,#12840,#7968,.T.);
#16335=EDGE_CURVE('',#12839,#12841,#7969,.T.);
#16336=EDGE_CURVE('',#12841,#12842,#7970,.T.);
#16337=EDGE_CURVE('',#12840,#12842,#7971,.T.);
#16338=EDGE_CURVE('',#12843,#12839,#7972,.T.);
#16339=EDGE_CURVE('',#12843,#12844,#7973,.T.);
#16340=EDGE_CURVE('',#12844,#12841,#7974,.T.);
#16341=EDGE_CURVE('',#12845,#12843,#7975,.T.);
#16342=EDGE_CURVE('',#12845,#12846,#7976,.T.);
#16343=EDGE_CURVE('',#12846,#12844,#7977,.T.);
#16344=EDGE_CURVE('',#12840,#12845,#7978,.T.);
#16345=EDGE_CURVE('',#12842,#12846,#7979,.T.);
#16346=EDGE_CURVE('',#12847,#12848,#7980,.T.);
#16347=EDGE_CURVE('',#12847,#12849,#7981,.T.);
#16348=EDGE_CURVE('',#12849,#12850,#7982,.T.);
#16349=EDGE_CURVE('',#12848,#12850,#7983,.T.);
#16350=EDGE_CURVE('',#12851,#12847,#7984,.T.);
#16351=EDGE_CURVE('',#12851,#12852,#7985,.T.);
#16352=EDGE_CURVE('',#12852,#12849,#7986,.T.);
#16353=EDGE_CURVE('',#12853,#12851,#7987,.T.);
#16354=EDGE_CURVE('',#12853,#12854,#7988,.T.);
#16355=EDGE_CURVE('',#12854,#12852,#7989,.T.);
#16356=EDGE_CURVE('',#12848,#12853,#7990,.T.);
#16357=EDGE_CURVE('',#12850,#12854,#7991,.T.);
#16358=EDGE_CURVE('',#12855,#12855,#2457,.T.);
#16359=EDGE_CURVE('',#12855,#12856,#7992,.T.);
#16360=EDGE_CURVE('',#12856,#12856,#2458,.T.);
#16361=EDGE_CURVE('',#12857,#12857,#2459,.T.);
#16362=EDGE_CURVE('',#12858,#12858,#2460,.T.);
#16363=EDGE_CURVE('',#12858,#12857,#7993,.T.);
#16364=EDGE_CURVE('',#12859,#12859,#2461,.T.);
#16365=EDGE_CURVE('',#12859,#12858,#7994,.T.);
#16366=EDGE_CURVE('',#12860,#12860,#2462,.T.);
#16367=EDGE_CURVE('',#12861,#12861,#2463,.T.);
#16368=EDGE_CURVE('',#12861,#12860,#7995,.T.);
#16369=EDGE_CURVE('',#12862,#12862,#2464,.T.);
#16370=EDGE_CURVE('',#12862,#12861,#7996,.T.);
#22583=ORIENTED_EDGE('',*,*,#16175,.F.);
#22584=ORIENTED_EDGE('',*,*,#16176,.T.);
#22585=ORIENTED_EDGE('',*,*,#16177,.T.);
#22586=ORIENTED_EDGE('',*,*,#16176,.F.);
#22587=ORIENTED_EDGE('',*,*,#16177,.F.);
#22588=ORIENTED_EDGE('',*,*,#16178,.T.);
#22589=ORIENTED_EDGE('',*,*,#16179,.T.);
#22590=ORIENTED_EDGE('',*,*,#16180,.T.);
#22591=ORIENTED_EDGE('',*,*,#16181,.T.);
#22592=ORIENTED_EDGE('',*,*,#16182,.T.);
#22593=ORIENTED_EDGE('',*,*,#16183,.T.);
#22594=ORIENTED_EDGE('',*,*,#16184,.F.);
#22595=ORIENTED_EDGE('',*,*,#16185,.T.);
#22596=ORIENTED_EDGE('',*,*,#16186,.T.);
#22597=ORIENTED_EDGE('',*,*,#16183,.F.);
#22598=ORIENTED_EDGE('',*,*,#16187,.F.);
#22599=ORIENTED_EDGE('',*,*,#16188,.T.);
#22600=ORIENTED_EDGE('',*,*,#16187,.T.);
#22601=ORIENTED_EDGE('',*,*,#16182,.F.);
#22602=ORIENTED_EDGE('',*,*,#16189,.F.);
#22603=ORIENTED_EDGE('',*,*,#16190,.T.);
#22604=ORIENTED_EDGE('',*,*,#16189,.T.);
#22605=ORIENTED_EDGE('',*,*,#16181,.F.);
#22606=ORIENTED_EDGE('',*,*,#16191,.F.);
#22607=ORIENTED_EDGE('',*,*,#16192,.T.);
#22608=ORIENTED_EDGE('',*,*,#16191,.T.);
#22609=ORIENTED_EDGE('',*,*,#16180,.F.);
#22610=ORIENTED_EDGE('',*,*,#16193,.F.);
#22611=ORIENTED_EDGE('',*,*,#16194,.T.);
#22612=ORIENTED_EDGE('',*,*,#16193,.T.);
#22613=ORIENTED_EDGE('',*,*,#16179,.F.);
#22614=ORIENTED_EDGE('',*,*,#16195,.F.);
#22615=ORIENTED_EDGE('',*,*,#16196,.T.);
#22616=ORIENTED_EDGE('',*,*,#16195,.T.);
#22617=ORIENTED_EDGE('',*,*,#16178,.F.);
#22618=ORIENTED_EDGE('',*,*,#16186,.F.);
#22619=ORIENTED_EDGE('',*,*,#16196,.F.);
#22620=ORIENTED_EDGE('',*,*,#16185,.F.);
#22621=ORIENTED_EDGE('',*,*,#16188,.F.);
#22622=ORIENTED_EDGE('',*,*,#16190,.F.);
#22623=ORIENTED_EDGE('',*,*,#16192,.F.);
#22624=ORIENTED_EDGE('',*,*,#16194,.F.);
#22625=ORIENTED_EDGE('',*,*,#16175,.T.);
#22626=ORIENTED_EDGE('',*,*,#16197,.F.);
#22627=ORIENTED_EDGE('',*,*,#16198,.T.);
#22628=ORIENTED_EDGE('',*,*,#16199,.F.);
#22629=ORIENTED_EDGE('',*,*,#16200,.T.);
#22630=ORIENTED_EDGE('',*,*,#16201,.T.);
#22631=ORIENTED_EDGE('',*,*,#16202,.F.);
#22632=ORIENTED_EDGE('',*,*,#16201,.F.);
#22633=ORIENTED_EDGE('',*,*,#16203,.T.);
#22634=ORIENTED_EDGE('',*,*,#16184,.T.);
#22635=ORIENTED_EDGE('',*,*,#16203,.F.);
#22636=ORIENTED_EDGE('',*,*,#16200,.F.);
#22637=ORIENTED_EDGE('',*,*,#16204,.F.);
#22638=ORIENTED_EDGE('',*,*,#16198,.F.);
#22639=ORIENTED_EDGE('',*,*,#16205,.F.);
#22640=ORIENTED_EDGE('',*,*,#16206,.T.);
#22641=ORIENTED_EDGE('',*,*,#16207,.F.);
#22642=ORIENTED_EDGE('',*,*,#16208,.F.);
#22643=ORIENTED_EDGE('',*,*,#16209,.F.);
#22644=ORIENTED_EDGE('',*,*,#16208,.T.);
#22645=ORIENTED_EDGE('',*,*,#16210,.F.);
#22646=ORIENTED_EDGE('',*,*,#16211,.F.);
#22647=ORIENTED_EDGE('',*,*,#16212,.F.);
#22648=ORIENTED_EDGE('',*,*,#16211,.T.);
#22649=ORIENTED_EDGE('',*,*,#16213,.F.);
#22650=ORIENTED_EDGE('',*,*,#16214,.F.);
#22651=ORIENTED_EDGE('',*,*,#16215,.F.);
#22652=ORIENTED_EDGE('',*,*,#16214,.T.);
#22653=ORIENTED_EDGE('',*,*,#16216,.F.);
#22654=ORIENTED_EDGE('',*,*,#16217,.F.);
#22655=ORIENTED_EDGE('',*,*,#16218,.F.);
#22656=ORIENTED_EDGE('',*,*,#16217,.T.);
#22657=ORIENTED_EDGE('',*,*,#16219,.F.);
#22658=ORIENTED_EDGE('',*,*,#16220,.F.);
#22659=ORIENTED_EDGE('',*,*,#16221,.F.);
#22660=ORIENTED_EDGE('',*,*,#16220,.T.);
#22661=ORIENTED_EDGE('',*,*,#16222,.F.);
#22662=ORIENTED_EDGE('',*,*,#16223,.F.);
#22663=ORIENTED_EDGE('',*,*,#16224,.F.);
#22664=ORIENTED_EDGE('',*,*,#16223,.T.);
#22665=ORIENTED_EDGE('',*,*,#16225,.F.);
#22666=ORIENTED_EDGE('',*,*,#16206,.F.);
#22667=ORIENTED_EDGE('',*,*,#16225,.T.);
#22668=ORIENTED_EDGE('',*,*,#16222,.T.);
#22669=ORIENTED_EDGE('',*,*,#16219,.T.);
#22670=ORIENTED_EDGE('',*,*,#16216,.T.);
#22671=ORIENTED_EDGE('',*,*,#16213,.T.);
#22672=ORIENTED_EDGE('',*,*,#16210,.T.);
#22673=ORIENTED_EDGE('',*,*,#16207,.T.);
#22674=ORIENTED_EDGE('',*,*,#16226,.F.);
#22675=ORIENTED_EDGE('',*,*,#16227,.T.);
#22676=ORIENTED_EDGE('',*,*,#16228,.T.);
#22677=ORIENTED_EDGE('',*,*,#16229,.F.);
#22678=ORIENTED_EDGE('',*,*,#16230,.F.);
#22679=ORIENTED_EDGE('',*,*,#16231,.T.);
#22680=ORIENTED_EDGE('',*,*,#16232,.T.);
#22681=ORIENTED_EDGE('',*,*,#16227,.F.);
#22682=ORIENTED_EDGE('',*,*,#16233,.F.);
#22683=ORIENTED_EDGE('',*,*,#16234,.T.);
#22684=ORIENTED_EDGE('',*,*,#16235,.T.);
#22685=ORIENTED_EDGE('',*,*,#16231,.F.);
#22686=ORIENTED_EDGE('',*,*,#16236,.F.);
#22687=ORIENTED_EDGE('',*,*,#16229,.T.);
#22688=ORIENTED_EDGE('',*,*,#16237,.T.);
#22689=ORIENTED_EDGE('',*,*,#16234,.F.);
#22690=ORIENTED_EDGE('',*,*,#16237,.F.);
#22691=ORIENTED_EDGE('',*,*,#16228,.F.);
#22692=ORIENTED_EDGE('',*,*,#16232,.F.);
#22693=ORIENTED_EDGE('',*,*,#16235,.F.);
#22694=ORIENTED_EDGE('',*,*,#16238,.F.);
#22695=ORIENTED_EDGE('',*,*,#16239,.T.);
#22696=ORIENTED_EDGE('',*,*,#16240,.T.);
#22697=ORIENTED_EDGE('',*,*,#16241,.F.);
#22698=ORIENTED_EDGE('',*,*,#16242,.F.);
#22699=ORIENTED_EDGE('',*,*,#16243,.T.);
#22700=ORIENTED_EDGE('',*,*,#16244,.T.);
#22701=ORIENTED_EDGE('',*,*,#16239,.F.);
#22702=ORIENTED_EDGE('',*,*,#16245,.F.);
#22703=ORIENTED_EDGE('',*,*,#16246,.T.);
#22704=ORIENTED_EDGE('',*,*,#16247,.T.);
#22705=ORIENTED_EDGE('',*,*,#16243,.F.);
#22706=ORIENTED_EDGE('',*,*,#16248,.F.);
#22707=ORIENTED_EDGE('',*,*,#16241,.T.);
#22708=ORIENTED_EDGE('',*,*,#16249,.T.);
#22709=ORIENTED_EDGE('',*,*,#16246,.F.);
#22710=ORIENTED_EDGE('',*,*,#16249,.F.);
#22711=ORIENTED_EDGE('',*,*,#16240,.F.);
#22712=ORIENTED_EDGE('',*,*,#16244,.F.);
#22713=ORIENTED_EDGE('',*,*,#16247,.F.);
#22714=ORIENTED_EDGE('',*,*,#16250,.F.);
#22715=ORIENTED_EDGE('',*,*,#16251,.T.);
#22716=ORIENTED_EDGE('',*,*,#16252,.T.);
#22717=ORIENTED_EDGE('',*,*,#16253,.F.);
#22718=ORIENTED_EDGE('',*,*,#16254,.F.);
#22719=ORIENTED_EDGE('',*,*,#16255,.T.);
#22720=ORIENTED_EDGE('',*,*,#16256,.T.);
#22721=ORIENTED_EDGE('',*,*,#16251,.F.);
#22722=ORIENTED_EDGE('',*,*,#16257,.F.);
#22723=ORIENTED_EDGE('',*,*,#16258,.T.);
#22724=ORIENTED_EDGE('',*,*,#16259,.T.);
#22725=ORIENTED_EDGE('',*,*,#16255,.F.);
#22726=ORIENTED_EDGE('',*,*,#16260,.F.);
#22727=ORIENTED_EDGE('',*,*,#16253,.T.);
#22728=ORIENTED_EDGE('',*,*,#16261,.T.);
#22729=ORIENTED_EDGE('',*,*,#16258,.F.);
#22730=ORIENTED_EDGE('',*,*,#16261,.F.);
#22731=ORIENTED_EDGE('',*,*,#16252,.F.);
#22732=ORIENTED_EDGE('',*,*,#16256,.F.);
#22733=ORIENTED_EDGE('',*,*,#16259,.F.);
#22734=ORIENTED_EDGE('',*,*,#16262,.F.);
#22735=ORIENTED_EDGE('',*,*,#16263,.T.);
#22736=ORIENTED_EDGE('',*,*,#16264,.T.);
#22737=ORIENTED_EDGE('',*,*,#16265,.F.);
#22738=ORIENTED_EDGE('',*,*,#16266,.F.);
#22739=ORIENTED_EDGE('',*,*,#16267,.T.);
#22740=ORIENTED_EDGE('',*,*,#16268,.T.);
#22741=ORIENTED_EDGE('',*,*,#16263,.F.);
#22742=ORIENTED_EDGE('',*,*,#16269,.F.);
#22743=ORIENTED_EDGE('',*,*,#16270,.T.);
#22744=ORIENTED_EDGE('',*,*,#16271,.T.);
#22745=ORIENTED_EDGE('',*,*,#16267,.F.);
#22746=ORIENTED_EDGE('',*,*,#16272,.F.);
#22747=ORIENTED_EDGE('',*,*,#16265,.T.);
#22748=ORIENTED_EDGE('',*,*,#16273,.T.);
#22749=ORIENTED_EDGE('',*,*,#16270,.F.);
#22750=ORIENTED_EDGE('',*,*,#16273,.F.);
#22751=ORIENTED_EDGE('',*,*,#16264,.F.);
#22752=ORIENTED_EDGE('',*,*,#16268,.F.);
#22753=ORIENTED_EDGE('',*,*,#16271,.F.);
#22754=ORIENTED_EDGE('',*,*,#16274,.F.);
#22755=ORIENTED_EDGE('',*,*,#16275,.T.);
#22756=ORIENTED_EDGE('',*,*,#16276,.T.);
#22757=ORIENTED_EDGE('',*,*,#16277,.F.);
#22758=ORIENTED_EDGE('',*,*,#16278,.F.);
#22759=ORIENTED_EDGE('',*,*,#16279,.T.);
#22760=ORIENTED_EDGE('',*,*,#16280,.T.);
#22761=ORIENTED_EDGE('',*,*,#16275,.F.);
#22762=ORIENTED_EDGE('',*,*,#16281,.F.);
#22763=ORIENTED_EDGE('',*,*,#16282,.T.);
#22764=ORIENTED_EDGE('',*,*,#16283,.T.);
#22765=ORIENTED_EDGE('',*,*,#16279,.F.);
#22766=ORIENTED_EDGE('',*,*,#16284,.F.);
#22767=ORIENTED_EDGE('',*,*,#16277,.T.);
#22768=ORIENTED_EDGE('',*,*,#16285,.T.);
#22769=ORIENTED_EDGE('',*,*,#16282,.F.);
#22770=ORIENTED_EDGE('',*,*,#16285,.F.);
#22771=ORIENTED_EDGE('',*,*,#16276,.F.);
#22772=ORIENTED_EDGE('',*,*,#16280,.F.);
#22773=ORIENTED_EDGE('',*,*,#16283,.F.);
#22774=ORIENTED_EDGE('',*,*,#16286,.F.);
#22775=ORIENTED_EDGE('',*,*,#16287,.T.);
#22776=ORIENTED_EDGE('',*,*,#16288,.T.);
#22777=ORIENTED_EDGE('',*,*,#16289,.F.);
#22778=ORIENTED_EDGE('',*,*,#16290,.F.);
#22779=ORIENTED_EDGE('',*,*,#16291,.T.);
#22780=ORIENTED_EDGE('',*,*,#16292,.T.);
#22781=ORIENTED_EDGE('',*,*,#16287,.F.);
#22782=ORIENTED_EDGE('',*,*,#16293,.F.);
#22783=ORIENTED_EDGE('',*,*,#16294,.T.);
#22784=ORIENTED_EDGE('',*,*,#16295,.T.);
#22785=ORIENTED_EDGE('',*,*,#16291,.F.);
#22786=ORIENTED_EDGE('',*,*,#16296,.F.);
#22787=ORIENTED_EDGE('',*,*,#16289,.T.);
#22788=ORIENTED_EDGE('',*,*,#16297,.T.);
#22789=ORIENTED_EDGE('',*,*,#16294,.F.);
#22790=ORIENTED_EDGE('',*,*,#16297,.F.);
#22791=ORIENTED_EDGE('',*,*,#16288,.F.);
#22792=ORIENTED_EDGE('',*,*,#16292,.F.);
#22793=ORIENTED_EDGE('',*,*,#16295,.F.);
#22794=ORIENTED_EDGE('',*,*,#16298,.F.);
#22795=ORIENTED_EDGE('',*,*,#16299,.T.);
#22796=ORIENTED_EDGE('',*,*,#16300,.T.);
#22797=ORIENTED_EDGE('',*,*,#16301,.F.);
#22798=ORIENTED_EDGE('',*,*,#16302,.F.);
#22799=ORIENTED_EDGE('',*,*,#16303,.T.);
#22800=ORIENTED_EDGE('',*,*,#16304,.T.);
#22801=ORIENTED_EDGE('',*,*,#16299,.F.);
#22802=ORIENTED_EDGE('',*,*,#16305,.F.);
#22803=ORIENTED_EDGE('',*,*,#16306,.T.);
#22804=ORIENTED_EDGE('',*,*,#16307,.T.);
#22805=ORIENTED_EDGE('',*,*,#16303,.F.);
#22806=ORIENTED_EDGE('',*,*,#16308,.F.);
#22807=ORIENTED_EDGE('',*,*,#16301,.T.);
#22808=ORIENTED_EDGE('',*,*,#16309,.T.);
#22809=ORIENTED_EDGE('',*,*,#16306,.F.);
#22810=ORIENTED_EDGE('',*,*,#16309,.F.);
#22811=ORIENTED_EDGE('',*,*,#16300,.F.);
#22812=ORIENTED_EDGE('',*,*,#16304,.F.);
#22813=ORIENTED_EDGE('',*,*,#16307,.F.);
#22814=ORIENTED_EDGE('',*,*,#16310,.F.);
#22815=ORIENTED_EDGE('',*,*,#16311,.T.);
#22816=ORIENTED_EDGE('',*,*,#16312,.T.);
#22817=ORIENTED_EDGE('',*,*,#16313,.F.);
#22818=ORIENTED_EDGE('',*,*,#16314,.F.);
#22819=ORIENTED_EDGE('',*,*,#16315,.T.);
#22820=ORIENTED_EDGE('',*,*,#16316,.T.);
#22821=ORIENTED_EDGE('',*,*,#16311,.F.);
#22822=ORIENTED_EDGE('',*,*,#16317,.F.);
#22823=ORIENTED_EDGE('',*,*,#16318,.T.);
#22824=ORIENTED_EDGE('',*,*,#16319,.T.);
#22825=ORIENTED_EDGE('',*,*,#16315,.F.);
#22826=ORIENTED_EDGE('',*,*,#16320,.F.);
#22827=ORIENTED_EDGE('',*,*,#16313,.T.);
#22828=ORIENTED_EDGE('',*,*,#16321,.T.);
#22829=ORIENTED_EDGE('',*,*,#16318,.F.);
#22830=ORIENTED_EDGE('',*,*,#16321,.F.);
#22831=ORIENTED_EDGE('',*,*,#16312,.F.);
#22832=ORIENTED_EDGE('',*,*,#16316,.F.);
#22833=ORIENTED_EDGE('',*,*,#16319,.F.);
#22834=ORIENTED_EDGE('',*,*,#16322,.F.);
#22835=ORIENTED_EDGE('',*,*,#16323,.T.);
#22836=ORIENTED_EDGE('',*,*,#16324,.T.);
#22837=ORIENTED_EDGE('',*,*,#16325,.F.);
#22838=ORIENTED_EDGE('',*,*,#16326,.F.);
#22839=ORIENTED_EDGE('',*,*,#16327,.T.);
#22840=ORIENTED_EDGE('',*,*,#16328,.T.);
#22841=ORIENTED_EDGE('',*,*,#16323,.F.);
#22842=ORIENTED_EDGE('',*,*,#16329,.F.);
#22843=ORIENTED_EDGE('',*,*,#16330,.T.);
#22844=ORIENTED_EDGE('',*,*,#16331,.T.);
#22845=ORIENTED_EDGE('',*,*,#16327,.F.);
#22846=ORIENTED_EDGE('',*,*,#16332,.F.);
#22847=ORIENTED_EDGE('',*,*,#16325,.T.);
#22848=ORIENTED_EDGE('',*,*,#16333,.T.);
#22849=ORIENTED_EDGE('',*,*,#16330,.F.);
#22850=ORIENTED_EDGE('',*,*,#16333,.F.);
#22851=ORIENTED_EDGE('',*,*,#16324,.F.);
#22852=ORIENTED_EDGE('',*,*,#16328,.F.);
#22853=ORIENTED_EDGE('',*,*,#16331,.F.);
#22854=ORIENTED_EDGE('',*,*,#16334,.F.);
#22855=ORIENTED_EDGE('',*,*,#16335,.T.);
#22856=ORIENTED_EDGE('',*,*,#16336,.T.);
#22857=ORIENTED_EDGE('',*,*,#16337,.F.);
#22858=ORIENTED_EDGE('',*,*,#16338,.F.);
#22859=ORIENTED_EDGE('',*,*,#16339,.T.);
#22860=ORIENTED_EDGE('',*,*,#16340,.T.);
#22861=ORIENTED_EDGE('',*,*,#16335,.F.);
#22862=ORIENTED_EDGE('',*,*,#16341,.F.);
#22863=ORIENTED_EDGE('',*,*,#16342,.T.);
#22864=ORIENTED_EDGE('',*,*,#16343,.T.);
#22865=ORIENTED_EDGE('',*,*,#16339,.F.);
#22866=ORIENTED_EDGE('',*,*,#16344,.F.);
#22867=ORIENTED_EDGE('',*,*,#16337,.T.);
#22868=ORIENTED_EDGE('',*,*,#16345,.T.);
#22869=ORIENTED_EDGE('',*,*,#16342,.F.);
#22870=ORIENTED_EDGE('',*,*,#16345,.F.);
#22871=ORIENTED_EDGE('',*,*,#16336,.F.);
#22872=ORIENTED_EDGE('',*,*,#16340,.F.);
#22873=ORIENTED_EDGE('',*,*,#16343,.F.);
#22874=ORIENTED_EDGE('',*,*,#16346,.F.);
#22875=ORIENTED_EDGE('',*,*,#16347,.T.);
#22876=ORIENTED_EDGE('',*,*,#16348,.T.);
#22877=ORIENTED_EDGE('',*,*,#16349,.F.);
#22878=ORIENTED_EDGE('',*,*,#16350,.F.);
#22879=ORIENTED_EDGE('',*,*,#16351,.T.);
#22880=ORIENTED_EDGE('',*,*,#16352,.T.);
#22881=ORIENTED_EDGE('',*,*,#16347,.F.);
#22882=ORIENTED_EDGE('',*,*,#16353,.F.);
#22883=ORIENTED_EDGE('',*,*,#16354,.T.);
#22884=ORIENTED_EDGE('',*,*,#16355,.T.);
#22885=ORIENTED_EDGE('',*,*,#16351,.F.);
#22886=ORIENTED_EDGE('',*,*,#16356,.F.);
#22887=ORIENTED_EDGE('',*,*,#16349,.T.);
#22888=ORIENTED_EDGE('',*,*,#16357,.T.);
#22889=ORIENTED_EDGE('',*,*,#16354,.F.);
#22890=ORIENTED_EDGE('',*,*,#16357,.F.);
#22891=ORIENTED_EDGE('',*,*,#16348,.F.);
#22892=ORIENTED_EDGE('',*,*,#16352,.F.);
#22893=ORIENTED_EDGE('',*,*,#16355,.F.);
#22894=ORIENTED_EDGE('',*,*,#16358,.T.);
#22895=ORIENTED_EDGE('',*,*,#16226,.T.);
#22896=ORIENTED_EDGE('',*,*,#16236,.T.);
#22897=ORIENTED_EDGE('',*,*,#16233,.T.);
#22898=ORIENTED_EDGE('',*,*,#16230,.T.);
#22899=ORIENTED_EDGE('',*,*,#16238,.T.);
#22900=ORIENTED_EDGE('',*,*,#16248,.T.);
#22901=ORIENTED_EDGE('',*,*,#16245,.T.);
#22902=ORIENTED_EDGE('',*,*,#16242,.T.);
#22903=ORIENTED_EDGE('',*,*,#16250,.T.);
#22904=ORIENTED_EDGE('',*,*,#16260,.T.);
#22905=ORIENTED_EDGE('',*,*,#16257,.T.);
#22906=ORIENTED_EDGE('',*,*,#16254,.T.);
#22907=ORIENTED_EDGE('',*,*,#16262,.T.);
#22908=ORIENTED_EDGE('',*,*,#16272,.T.);
#22909=ORIENTED_EDGE('',*,*,#16269,.T.);
#22910=ORIENTED_EDGE('',*,*,#16266,.T.);
#22911=ORIENTED_EDGE('',*,*,#16274,.T.);
#22912=ORIENTED_EDGE('',*,*,#16284,.T.);
#22913=ORIENTED_EDGE('',*,*,#16281,.T.);
#22914=ORIENTED_EDGE('',*,*,#16278,.T.);
#22915=ORIENTED_EDGE('',*,*,#16286,.T.);
#22916=ORIENTED_EDGE('',*,*,#16296,.T.);
#22917=ORIENTED_EDGE('',*,*,#16293,.T.);
#22918=ORIENTED_EDGE('',*,*,#16290,.T.);
#22919=ORIENTED_EDGE('',*,*,#16298,.T.);
#22920=ORIENTED_EDGE('',*,*,#16308,.T.);
#22921=ORIENTED_EDGE('',*,*,#16305,.T.);
#22922=ORIENTED_EDGE('',*,*,#16302,.T.);
#22923=ORIENTED_EDGE('',*,*,#16310,.T.);
#22924=ORIENTED_EDGE('',*,*,#16320,.T.);
#22925=ORIENTED_EDGE('',*,*,#16317,.T.);
#22926=ORIENTED_EDGE('',*,*,#16314,.T.);
#22927=ORIENTED_EDGE('',*,*,#16322,.T.);
#22928=ORIENTED_EDGE('',*,*,#16332,.T.);
#22929=ORIENTED_EDGE('',*,*,#16329,.T.);
#22930=ORIENTED_EDGE('',*,*,#16326,.T.);
#22931=ORIENTED_EDGE('',*,*,#16334,.T.);
#22932=ORIENTED_EDGE('',*,*,#16344,.T.);
#22933=ORIENTED_EDGE('',*,*,#16341,.T.);
#22934=ORIENTED_EDGE('',*,*,#16338,.T.);
#22935=ORIENTED_EDGE('',*,*,#16346,.T.);
#22936=ORIENTED_EDGE('',*,*,#16356,.T.);
#22937=ORIENTED_EDGE('',*,*,#16353,.T.);
#22938=ORIENTED_EDGE('',*,*,#16350,.T.);
#22939=ORIENTED_EDGE('',*,*,#16205,.T.);
#22940=ORIENTED_EDGE('',*,*,#16209,.T.);
#22941=ORIENTED_EDGE('',*,*,#16212,.T.);
#22942=ORIENTED_EDGE('',*,*,#16215,.T.);
#22943=ORIENTED_EDGE('',*,*,#16218,.T.);
#22944=ORIENTED_EDGE('',*,*,#16221,.T.);
#22945=ORIENTED_EDGE('',*,*,#16224,.T.);
#22946=ORIENTED_EDGE('',*,*,#16358,.F.);
#22947=ORIENTED_EDGE('',*,*,#16359,.T.);
#22948=ORIENTED_EDGE('',*,*,#16360,.F.);
#22949=ORIENTED_EDGE('',*,*,#16359,.F.);
#22950=ORIENTED_EDGE('',*,*,#16361,.F.);
#22951=ORIENTED_EDGE('',*,*,#16362,.F.);
#22952=ORIENTED_EDGE('',*,*,#16363,.T.);
#22953=ORIENTED_EDGE('',*,*,#16361,.T.);
#22954=ORIENTED_EDGE('',*,*,#16363,.F.);
#22955=ORIENTED_EDGE('',*,*,#16364,.F.);
#22956=ORIENTED_EDGE('',*,*,#16365,.T.);
#22957=ORIENTED_EDGE('',*,*,#16362,.T.);
#22958=ORIENTED_EDGE('',*,*,#16365,.F.);
#22959=ORIENTED_EDGE('',*,*,#16204,.T.);
#22960=ORIENTED_EDGE('',*,*,#16199,.T.);
#22961=ORIENTED_EDGE('',*,*,#16202,.T.);
#22962=ORIENTED_EDGE('',*,*,#16197,.T.);
#22963=ORIENTED_EDGE('',*,*,#16366,.F.);
#22964=ORIENTED_EDGE('',*,*,#16364,.T.);
#22965=ORIENTED_EDGE('',*,*,#16367,.F.);
#22966=ORIENTED_EDGE('',*,*,#16368,.T.);
#22967=ORIENTED_EDGE('',*,*,#16366,.T.);
#22968=ORIENTED_EDGE('',*,*,#16368,.F.);
#22969=ORIENTED_EDGE('',*,*,#16369,.F.);
#22970=ORIENTED_EDGE('',*,*,#16370,.T.);
#22971=ORIENTED_EDGE('',*,*,#16367,.T.);
#22972=ORIENTED_EDGE('',*,*,#16370,.F.);
#22973=ORIENTED_EDGE('',*,*,#16369,.T.);
#22974=ORIENTED_EDGE('',*,*,#16360,.T.);
#26593=PLANE('',#29882);
#26594=PLANE('',#29883);
#26595=PLANE('',#29885);
#26596=PLANE('',#29886);
#26597=PLANE('',#29887);
#26598=PLANE('',#29888);
#26599=PLANE('',#29889);
#26600=PLANE('',#29890);
#26601=PLANE('',#29891);
#26602=PLANE('',#29892);
#26603=PLANE('',#29894);
#26604=PLANE('',#29901);
#26605=PLANE('',#29902);
#26606=PLANE('',#29903);
#26607=PLANE('',#29907);
#26608=PLANE('',#29908);
#26609=PLANE('',#29909);
#26610=PLANE('',#29910);
#26611=PLANE('',#29911);
#26612=PLANE('',#29912);
#26613=PLANE('',#29913);
#26614=PLANE('',#29914);
#26615=PLANE('',#29915);
#26616=PLANE('',#29916);
#26617=PLANE('',#29917);
#26618=PLANE('',#29918);
#26619=PLANE('',#29919);
#26620=PLANE('',#29920);
#26621=PLANE('',#29921);
#26622=PLANE('',#29922);
#26623=PLANE('',#29923);
#26624=PLANE('',#29924);
#26625=PLANE('',#29925);
#26626=PLANE('',#29926);
#26627=PLANE('',#29927);
#26628=PLANE('',#29928);
#26629=PLANE('',#29929);
#26630=PLANE('',#29930);
#26631=PLANE('',#29931);
#26632=PLANE('',#29932);
#26633=PLANE('',#29933);
#26634=PLANE('',#29934);
#26635=PLANE('',#29935);
#26636=PLANE('',#29936);
#26637=PLANE('',#29937);
#26638=PLANE('',#29938);
#26639=PLANE('',#29939);
#26640=PLANE('',#29940);
#26641=PLANE('',#29941);
#26642=PLANE('',#29942);
#26643=PLANE('',#29943);
#26644=PLANE('',#29944);
#26645=PLANE('',#29945);
#26646=PLANE('',#29946);
#26647=PLANE('',#29947);
#26648=PLANE('',#29948);
#26649=PLANE('',#29949);
#26650=PLANE('',#29950);
#26651=PLANE('',#29951);
#26652=PLANE('',#29952);
#26653=PLANE('',#29953);
#26654=PLANE('',#29954);
#26655=PLANE('',#29955);
#26656=PLANE('',#29956);
#26657=PLANE('',#29957);
#26658=PLANE('',#29958);
#26659=PLANE('',#29959);
#26660=PLANE('',#29960);
#26661=PLANE('',#29961);
#26662=PLANE('',#29962);
#26663=PLANE('',#29963);
#26664=PLANE('',#29964);
#26665=PLANE('',#29965);
#26666=PLANE('',#29969);
#26667=PLANE('',#29975);
#26668=PLANE('',#29981);
#27769=ADVANCED_FACE('',(#3861),#1661,.T.);
#27770=ADVANCED_FACE('',(#3862),#26593,.F.);
#27771=ADVANCED_FACE('',(#3863,#1931),#26594,.T.);
#27772=ADVANCED_FACE('',(#3864),#26595,.T.);
#27773=ADVANCED_FACE('',(#3865),#26596,.T.);
#27774=ADVANCED_FACE('',(#3866),#26597,.T.);
#27775=ADVANCED_FACE('',(#3867),#26598,.T.);
#27776=ADVANCED_FACE('',(#3868),#26599,.T.);
#27777=ADVANCED_FACE('',(#3869),#26600,.T.);
#27778=ADVANCED_FACE('',(#3870,#1932),#26601,.F.);
#27779=ADVANCED_FACE('',(#3871),#26602,.T.);
#27780=ADVANCED_FACE('',(#3872),#26603,.T.);
#27781=ADVANCED_FACE('',(#3873),#1662,.T.);
#27782=ADVANCED_FACE('',(#3874),#1663,.T.);
#27783=ADVANCED_FACE('',(#3875),#26604,.T.);
#27784=ADVANCED_FACE('',(#3876),#26605,.T.);
#27785=ADVANCED_FACE('',(#3877),#26606,.T.);
#27786=ADVANCED_FACE('',(#3878),#1664,.T.);
#27787=ADVANCED_FACE('',(#3879),#26607,.T.);
#27788=ADVANCED_FACE('',(#3880),#26608,.T.);
#27789=ADVANCED_FACE('',(#3881),#26609,.F.);
#27790=ADVANCED_FACE('',(#3882),#26610,.F.);
#27791=ADVANCED_FACE('',(#3883),#26611,.F.);
#27792=ADVANCED_FACE('',(#3884),#26612,.F.);
#27793=ADVANCED_FACE('',(#3885),#26613,.F.);
#27794=ADVANCED_FACE('',(#3886),#26614,.F.);
#27795=ADVANCED_FACE('',(#3887),#26615,.F.);
#27796=ADVANCED_FACE('',(#3888),#26616,.F.);
#27797=ADVANCED_FACE('',(#3889),#26617,.F.);
#27798=ADVANCED_FACE('',(#3890),#26618,.F.);
#27799=ADVANCED_FACE('',(#3891),#26619,.F.);
#27800=ADVANCED_FACE('',(#3892),#26620,.F.);
#27801=ADVANCED_FACE('',(#3893),#26621,.F.);
#27802=ADVANCED_FACE('',(#3894),#26622,.F.);
#27803=ADVANCED_FACE('',(#3895),#26623,.F.);
#27804=ADVANCED_FACE('',(#3896),#26624,.F.);
#27805=ADVANCED_FACE('',(#3897),#26625,.F.);
#27806=ADVANCED_FACE('',(#3898),#26626,.F.);
#27807=ADVANCED_FACE('',(#3899),#26627,.F.);
#27808=ADVANCED_FACE('',(#3900),#26628,.F.);
#27809=ADVANCED_FACE('',(#3901),#26629,.F.);
#27810=ADVANCED_FACE('',(#3902),#26630,.F.);
#27811=ADVANCED_FACE('',(#3903),#26631,.F.);
#27812=ADVANCED_FACE('',(#3904),#26632,.F.);
#27813=ADVANCED_FACE('',(#3905),#26633,.F.);
#27814=ADVANCED_FACE('',(#3906),#26634,.F.);
#27815=ADVANCED_FACE('',(#3907),#26635,.F.);
#27816=ADVANCED_FACE('',(#3908),#26636,.F.);
#27817=ADVANCED_FACE('',(#3909),#26637,.F.);
#27818=ADVANCED_FACE('',(#3910),#26638,.F.);
#27819=ADVANCED_FACE('',(#3911),#26639,.F.);
#27820=ADVANCED_FACE('',(#3912),#26640,.F.);
#27821=ADVANCED_FACE('',(#3913),#26641,.F.);
#27822=ADVANCED_FACE('',(#3914),#26642,.F.);
#27823=ADVANCED_FACE('',(#3915),#26643,.F.);
#27824=ADVANCED_FACE('',(#3916),#26644,.F.);
#27825=ADVANCED_FACE('',(#3917),#26645,.F.);
#27826=ADVANCED_FACE('',(#3918),#26646,.F.);
#27827=ADVANCED_FACE('',(#3919),#26647,.F.);
#27828=ADVANCED_FACE('',(#3920),#26648,.F.);
#27829=ADVANCED_FACE('',(#3921),#26649,.F.);
#27830=ADVANCED_FACE('',(#3922),#26650,.F.);
#27831=ADVANCED_FACE('',(#3923),#26651,.F.);
#27832=ADVANCED_FACE('',(#3924),#26652,.F.);
#27833=ADVANCED_FACE('',(#3925),#26653,.F.);
#27834=ADVANCED_FACE('',(#3926),#26654,.F.);
#27835=ADVANCED_FACE('',(#3927),#26655,.F.);
#27836=ADVANCED_FACE('',(#3928),#26656,.F.);
#27837=ADVANCED_FACE('',(#3929),#26657,.F.);
#27838=ADVANCED_FACE('',(#3930),#26658,.F.);
#27839=ADVANCED_FACE('',(#3931),#26659,.F.);
#27840=ADVANCED_FACE('',(#3932),#26660,.F.);
#27841=ADVANCED_FACE('',(#3933),#26661,.F.);
#27842=ADVANCED_FACE('',(#3934),#26662,.F.);
#27843=ADVANCED_FACE('',(#3935),#26663,.F.);
#27844=ADVANCED_FACE('',(#3936),#26664,.F.);
#27845=ADVANCED_FACE('',(#3937,#1933,#1934,#1935,#1936,#1937,#1938,#1939,
#1940,#1941,#1942,#1943,#1944),#26665,.F.);
#27846=ADVANCED_FACE('',(#3938),#1665,.F.);
#27847=ADVANCED_FACE('',(#3939),#26666,.T.);
#27848=ADVANCED_FACE('',(#3940),#2859,.T.);
#27849=ADVANCED_FACE('',(#3941,#1945),#1666,.T.);
#27850=ADVANCED_FACE('',(#3942,#1946),#26667,.T.);
#27851=ADVANCED_FACE('',(#3943),#1667,.T.);
#27852=ADVANCED_FACE('',(#3944),#2860,.T.);
#27853=ADVANCED_FACE('',(#3945,#1947),#26668,.T.);
#28466=CLOSED_SHELL('',(#27769,#27770,#27771,#27772,#27773,#27774,#27775,
#27776,#27777,#27778,#27779,#27780,#27781,#27782,#27783,#27784,#27785,#27786,
#27787,#27788,#27789,#27790,#27791,#27792,#27793,#27794,#27795,#27796,#27797,
#27798,#27799,#27800,#27801,#27802,#27803,#27804,#27805,#27806,#27807,#27808,
#27809,#27810,#27811,#27812,#27813,#27814,#27815,#27816,#27817,#27818,#27819,
#27820,#27821,#27822,#27823,#27824,#27825,#27826,#27827,#27828,#27829,#27830,
#27831,#27832,#27833,#27834,#27835,#27836,#27837,#27838,#27839,#27840,#27841,
#27842,#27843,#27844,#27845,#27846,#27847,#27848,#27849,#27850,#27851,#27852,
#27853));
#29878=AXIS2_PLACEMENT_3D('',#48688,#34754,#34755);
#29879=AXIS2_PLACEMENT_3D('',#48689,#34756,#34757);
#29880=AXIS2_PLACEMENT_3D('',#48691,#34758,#34759);
#29881=AXIS2_PLACEMENT_3D('',#48694,#34761,#34762);
#29882=AXIS2_PLACEMENT_3D('',#48695,#34763,#34764);
#29883=AXIS2_PLACEMENT_3D('',#48696,#34765,#34766);
#29884=AXIS2_PLACEMENT_3D('',#48710,#34773,#34774);
#29885=AXIS2_PLACEMENT_3D('',#48711,#34775,#34776);
#29886=AXIS2_PLACEMENT_3D('',#48717,#34780,#34781);
#29887=AXIS2_PLACEMENT_3D('',#48721,#34784,#34785);
#29888=AXIS2_PLACEMENT_3D('',#48725,#34788,#34789);
#29889=AXIS2_PLACEMENT_3D('',#48729,#34792,#34793);
#29890=AXIS2_PLACEMENT_3D('',#48733,#34796,#34797);
#29891=AXIS2_PLACEMENT_3D('',#48735,#34799,#34800);
#29892=AXIS2_PLACEMENT_3D('',#48736,#34801,#34802);
#29893=AXIS2_PLACEMENT_3D('',#48740,#34804,#34805);
#29894=AXIS2_PLACEMENT_3D('',#48741,#34806,#34807);
#29895=AXIS2_PLACEMENT_3D('',#48746,#34809,#34810);
#29896=AXIS2_PLACEMENT_3D('',#48747,#34811,#34812);
#29897=AXIS2_PLACEMENT_3D('',#48748,#34813,#34814);
#29898=AXIS2_PLACEMENT_3D('',#48786,#34816,#34817);
#29899=AXIS2_PLACEMENT_3D('',#48789,#34818,#34819);
#29900=AXIS2_PLACEMENT_3D('',#48793,#34821,#34822);
#29901=AXIS2_PLACEMENT_3D('',#48795,#34824,#34825);
#29902=AXIS2_PLACEMENT_3D('',#48801,#34829,#34830);
#29903=AXIS2_PLACEMENT_3D('',#48807,#34834,#34835);
#29904=AXIS2_PLACEMENT_3D('',#48813,#34839,#34840);
#29905=AXIS2_PLACEMENT_3D('',#48815,#34841,#34842);
#29906=AXIS2_PLACEMENT_3D('',#48817,#34843,#34844);
#29907=AXIS2_PLACEMENT_3D('',#48819,#34846,#34847);
#29908=AXIS2_PLACEMENT_3D('',#48825,#34851,#34852);
#29909=AXIS2_PLACEMENT_3D('',#48828,#34855,#34856);
#29910=AXIS2_PLACEMENT_3D('',#48829,#34857,#34858);
#29911=AXIS2_PLACEMENT_3D('',#48838,#34863,#34864);
#29912=AXIS2_PLACEMENT_3D('',#48844,#34868,#34869);
#29913=AXIS2_PLACEMENT_3D('',#48850,#34873,#34874);
#29914=AXIS2_PLACEMENT_3D('',#48853,#34877,#34878);
#29915=AXIS2_PLACEMENT_3D('',#48854,#34879,#34880);
#29916=AXIS2_PLACEMENT_3D('',#48863,#34885,#34886);
#29917=AXIS2_PLACEMENT_3D('',#48869,#34890,#34891);
#29918=AXIS2_PLACEMENT_3D('',#48875,#34895,#34896);
#29919=AXIS2_PLACEMENT_3D('',#48878,#34899,#34900);
#29920=AXIS2_PLACEMENT_3D('',#48879,#34901,#34902);
#29921=AXIS2_PLACEMENT_3D('',#48888,#34907,#34908);
#29922=AXIS2_PLACEMENT_3D('',#48894,#34912,#34913);
#29923=AXIS2_PLACEMENT_3D('',#48900,#34917,#34918);
#29924=AXIS2_PLACEMENT_3D('',#48903,#34921,#34922);
#29925=AXIS2_PLACEMENT_3D('',#48904,#34923,#34924);
#29926=AXIS2_PLACEMENT_3D('',#48913,#34929,#34930);
#29927=AXIS2_PLACEMENT_3D('',#48919,#34934,#34935);
#29928=AXIS2_PLACEMENT_3D('',#48925,#34939,#34940);
#29929=AXIS2_PLACEMENT_3D('',#48928,#34943,#34944);
#29930=AXIS2_PLACEMENT_3D('',#48929,#34945,#34946);
#29931=AXIS2_PLACEMENT_3D('',#48938,#34951,#34952);
#29932=AXIS2_PLACEMENT_3D('',#48944,#34956,#34957);
#29933=AXIS2_PLACEMENT_3D('',#48950,#34961,#34962);
#29934=AXIS2_PLACEMENT_3D('',#48953,#34965,#34966);
#29935=AXIS2_PLACEMENT_3D('',#48954,#34967,#34968);
#29936=AXIS2_PLACEMENT_3D('',#48963,#34973,#34974);
#29937=AXIS2_PLACEMENT_3D('',#48969,#34978,#34979);
#29938=AXIS2_PLACEMENT_3D('',#48975,#34983,#34984);
#29939=AXIS2_PLACEMENT_3D('',#48978,#34987,#34988);
#29940=AXIS2_PLACEMENT_3D('',#48979,#34989,#34990);
#29941=AXIS2_PLACEMENT_3D('',#48988,#34995,#34996);
#29942=AXIS2_PLACEMENT_3D('',#48994,#35000,#35001);
#29943=AXIS2_PLACEMENT_3D('',#49000,#35005,#35006);
#29944=AXIS2_PLACEMENT_3D('',#49003,#35009,#35010);
#29945=AXIS2_PLACEMENT_3D('',#49004,#35011,#35012);
#29946=AXIS2_PLACEMENT_3D('',#49013,#35017,#35018);
#29947=AXIS2_PLACEMENT_3D('',#49019,#35022,#35023);
#29948=AXIS2_PLACEMENT_3D('',#49025,#35027,#35028);
#29949=AXIS2_PLACEMENT_3D('',#49028,#35031,#35032);
#29950=AXIS2_PLACEMENT_3D('',#49029,#35033,#35034);
#29951=AXIS2_PLACEMENT_3D('',#49038,#35039,#35040);
#29952=AXIS2_PLACEMENT_3D('',#49044,#35044,#35045);
#29953=AXIS2_PLACEMENT_3D('',#49050,#35049,#35050);
#29954=AXIS2_PLACEMENT_3D('',#49053,#35053,#35054);
#29955=AXIS2_PLACEMENT_3D('',#49054,#35055,#35056);
#29956=AXIS2_PLACEMENT_3D('',#49063,#35061,#35062);
#29957=AXIS2_PLACEMENT_3D('',#49069,#35066,#35067);
#29958=AXIS2_PLACEMENT_3D('',#49075,#35071,#35072);
#29959=AXIS2_PLACEMENT_3D('',#49078,#35075,#35076);
#29960=AXIS2_PLACEMENT_3D('',#49079,#35077,#35078);
#29961=AXIS2_PLACEMENT_3D('',#49088,#35083,#35084);
#29962=AXIS2_PLACEMENT_3D('',#49094,#35088,#35089);
#29963=AXIS2_PLACEMENT_3D('',#49100,#35093,#35094);
#29964=AXIS2_PLACEMENT_3D('',#49103,#35097,#35098);
#29965=AXIS2_PLACEMENT_3D('',#49104,#35099,#35100);
#29966=AXIS2_PLACEMENT_3D('',#49106,#35101,#35102);
#29967=AXIS2_PLACEMENT_3D('',#49107,#35103,#35104);
#29968=AXIS2_PLACEMENT_3D('',#49110,#35106,#35107);
#29969=AXIS2_PLACEMENT_3D('',#49111,#35108,#35109);
#29970=AXIS2_PLACEMENT_3D('',#49113,#35110,#35111);
#29971=AXIS2_PLACEMENT_3D('',#49114,#35112,#35113);
#29972=AXIS2_PLACEMENT_3D('',#49116,#35114,#35115);
#29973=AXIS2_PLACEMENT_3D('',#49118,#35117,#35118);
#29974=AXIS2_PLACEMENT_3D('',#49120,#35119,#35120);
#29975=AXIS2_PLACEMENT_3D('',#49122,#35122,#35123);
#29976=AXIS2_PLACEMENT_3D('',#49124,#35124,#35125);
#29977=AXIS2_PLACEMENT_3D('',#49125,#35126,#35127);
#29978=AXIS2_PLACEMENT_3D('',#49127,#35128,#35129);
#29979=AXIS2_PLACEMENT_3D('',#49129,#35131,#35132);
#29980=AXIS2_PLACEMENT_3D('',#49131,#35133,#35134);
#29981=AXIS2_PLACEMENT_3D('',#49133,#35136,#35137);
#34754=DIRECTION('axis',(0.,0.,1.));
#34755=DIRECTION('refdir',(1.,0.,0.));
#34756=DIRECTION('center_axis',(0.,0.,1.));
#34757=DIRECTION('ref_axis',(1.,0.,0.));
#34758=DIRECTION('center_axis',(0.,0.,1.));
#34759=DIRECTION('ref_axis',(1.,0.,0.));
#34760=DIRECTION('',(0.,0.,-1.));
#34761=DIRECTION('center_axis',(0.,0.,1.));
#34762=DIRECTION('ref_axis',(1.,0.,0.));
#34763=DIRECTION('center_axis',(0.,0.,1.));
#34764=DIRECTION('ref_axis',(1.,0.,0.));
#34765=DIRECTION('center_axis',(0.,0.,1.));
#34766=DIRECTION('ref_axis',(1.,0.,0.));
#34767=DIRECTION('',(0.499999999999999,0.866025403784439,0.));
#34768=DIRECTION('',(-0.499999999999999,0.866025403784439,0.));
#34769=DIRECTION('',(-1.,1.37354477598826E-16,0.));
#34770=DIRECTION('',(-0.5,-0.866025403784439,0.));
#34771=DIRECTION('',(0.499999999999998,-0.86602540378444,0.));
#34772=DIRECTION('',(1.,-1.37354477598826E-16,0.));
#34773=DIRECTION('center_axis',(0.,0.,1.));
#34774=DIRECTION('ref_axis',(1.,0.,0.));
#34775=DIRECTION('center_axis',(-1.37354477598826E-16,-1.,0.));
#34776=DIRECTION('ref_axis',(1.,-1.37354477598826E-16,0.));
#34777=DIRECTION('',(1.,-1.37354477598826E-16,0.));
#34778=DIRECTION('',(0.,0.,1.));
#34779=DIRECTION('',(0.,0.,1.));
#34780=DIRECTION('center_axis',(-0.86602540378444,-0.499999999999998,0.));
#34781=DIRECTION('ref_axis',(0.499999999999998,-0.86602540378444,0.));
#34782=DIRECTION('',(0.499999999999998,-0.86602540378444,0.));
#34783=DIRECTION('',(0.,0.,1.));
#34784=DIRECTION('center_axis',(-0.866025403784439,0.5,0.));
#34785=DIRECTION('ref_axis',(-0.5,-0.866025403784439,0.));
#34786=DIRECTION('',(-0.5,-0.866025403784439,0.));
#34787=DIRECTION('',(0.,0.,1.));
#34788=DIRECTION('center_axis',(1.37354477598826E-16,1.,0.));
#34789=DIRECTION('ref_axis',(-1.,1.37354477598826E-16,0.));
#34790=DIRECTION('',(-1.,1.37354477598826E-16,0.));
#34791=DIRECTION('',(0.,0.,1.));
#34792=DIRECTION('center_axis',(0.866025403784439,0.499999999999999,0.));
#34793=DIRECTION('ref_axis',(-0.499999999999999,0.866025403784439,0.));
#34794=DIRECTION('',(-0.499999999999999,0.866025403784439,0.));
#34795=DIRECTION('',(0.,0.,1.));
#34796=DIRECTION('center_axis',(0.866025403784439,-0.499999999999999,0.));
#34797=DIRECTION('ref_axis',(0.499999999999999,0.866025403784439,0.));
#34798=DIRECTION('',(0.499999999999999,0.866025403784439,0.));
#34799=DIRECTION('center_axis',(0.,0.,1.));
#34800=DIRECTION('ref_axis',(1.,0.,0.));
#34801=DIRECTION('center_axis',(0.,0.,1.));
#34802=DIRECTION('ref_axis',(1.,0.,0.));
#34803=DIRECTION('',(0.,1.,0.));
#34804=DIRECTION('center_axis',(0.,0.,1.));
#34805=DIRECTION('ref_axis',(1.,0.,0.));
#34806=DIRECTION('center_axis',(0.,0.,1.));
#34807=DIRECTION('ref_axis',(1.,0.,0.));
#34808=DIRECTION('',(0.,-1.,0.));
#34809=DIRECTION('center_axis',(0.,0.,1.));
#34810=DIRECTION('ref_axis',(1.,0.,0.));
#34811=DIRECTION('center_axis',(0.,0.,1.));
#34812=DIRECTION('ref_axis',(1.,0.,0.));
#34813=DIRECTION('center_axis',(0.,0.,1.));
#34814=DIRECTION('ref_axis',(1.,0.,0.));
#34815=DIRECTION('',(0.,0.,-1.));
#34816=DIRECTION('center_axis',(0.,-1.,0.));
#34817=DIRECTION('ref_axis',(1.,0.,0.));
#34818=DIRECTION('center_axis',(0.,1.,0.));
#34819=DIRECTION('ref_axis',(1.,0.,0.));
#34820=DIRECTION('',(0.,-1.,0.));
#34821=DIRECTION('center_axis',(0.,-1.,0.));
#34822=DIRECTION('ref_axis',(1.,0.,0.));
#34823=DIRECTION('',(0.,-1.,0.));
#34824=DIRECTION('center_axis',(0.452956278458863,0.,0.89153273064128));
#34825=DIRECTION('ref_axis',(-0.89153273064128,0.,0.452956278458863));
#34826=DIRECTION('',(0.89153273064128,0.,-0.452956278458863));
#34827=DIRECTION('',(-0.89153273064128,0.,0.452956278458863));
#34828=DIRECTION('',(0.,-1.,0.));
#34829=DIRECTION('center_axis',(0.866025403784419,0.,-0.500000000000034));
#34830=DIRECTION('ref_axis',(0.500000000000034,0.,0.866025403784419));
#34831=DIRECTION('',(-0.500000000000034,0.,-0.866025403784419));
#34832=DIRECTION('',(0.500000000000034,0.,0.866025403784419));
#34833=DIRECTION('',(0.,-1.,0.));
#34834=DIRECTION('center_axis',(-0.54561185381123,0.,-0.838038009269671));
#34835=DIRECTION('ref_axis',(0.838038009269671,0.,-0.54561185381123));
#34836=DIRECTION('',(-0.838038009269671,0.,0.54561185381123));
#34837=DIRECTION('',(0.838038009269671,0.,-0.54561185381123));
#34838=DIRECTION('',(0.,-1.,0.));
#34839=DIRECTION('center_axis',(0.,-1.,0.));
#34840=DIRECTION('ref_axis',(-0.545611853811243,0.,-0.838038009269663));
#34841=DIRECTION('center_axis',(0.,1.,0.));
#34842=DIRECTION('ref_axis',(1.,0.,0.));
#34843=DIRECTION('center_axis',(0.,-1.,0.));
#34844=DIRECTION('ref_axis',(1.,0.,0.));
#34845=DIRECTION('',(0.,-1.,0.));
#34846=DIRECTION('center_axis',(-0.54561185381123,0.,-0.838038009269671));
#34847=DIRECTION('ref_axis',(0.838038009269671,0.,-0.54561185381123));
#34848=DIRECTION('',(-0.838038009269671,0.,0.54561185381123));
#34849=DIRECTION('',(0.838038009269671,0.,-0.54561185381123));
#34850=DIRECTION('',(0.,-1.,0.));
#34851=DIRECTION('center_axis',(0.452956278458863,0.,0.89153273064128));
#34852=DIRECTION('ref_axis',(-0.89153273064128,0.,0.452956278458863));
#34853=DIRECTION('',(0.89153273064128,0.,-0.452956278458863));
#34854=DIRECTION('',(-0.89153273064128,0.,0.452956278458863));
#34855=DIRECTION('center_axis',(0.,1.,0.));
#34856=DIRECTION('ref_axis',(1.,0.,0.));
#34857=DIRECTION('center_axis',(-0.309016994374968,0.,-0.951056516295147));
#34858=DIRECTION('ref_axis',(-0.951056516295147,0.,0.309016994374968));
#34859=DIRECTION('',(-0.951056516295147,0.,0.309016994374968));
#34860=DIRECTION('',(0.,1.,0.));
#34861=DIRECTION('',(-0.951056516295147,0.,0.309016994374968));
#34862=DIRECTION('',(0.,1.,0.));
#34863=DIRECTION('center_axis',(0.951056516295164,0.,-0.309016994374916));
#34864=DIRECTION('ref_axis',(-0.309016994374916,0.,-0.951056516295164));
#34865=DIRECTION('',(-0.309016994374916,0.,-0.951056516295164));
#34866=DIRECTION('',(0.,1.,0.));
#34867=DIRECTION('',(-0.309016994374916,0.,-0.951056516295164));
#34868=DIRECTION('center_axis',(0.30901699437493,0.,0.951056516295159));
#34869=DIRECTION('ref_axis',(0.951056516295159,0.,-0.30901699437493));
#34870=DIRECTION('',(0.951056516295159,0.,-0.30901699437493));
#34871=DIRECTION('',(0.,1.,0.));
#34872=DIRECTION('',(0.951056516295159,0.,-0.30901699437493));
#34873=DIRECTION('center_axis',(-0.951056516295155,0.,0.309016994374944));
#34874=DIRECTION('ref_axis',(0.309016994374944,0.,0.951056516295155));
#34875=DIRECTION('',(0.309016994374944,0.,0.951056516295155));
#34876=DIRECTION('',(0.309016994374944,0.,0.951056516295155));
#34877=DIRECTION('center_axis',(0.,1.,0.));
#34878=DIRECTION('ref_axis',(0.,0.,1.));
#34879=DIRECTION('center_axis',(0.587785252292488,0.,-0.809016994374936));
#34880=DIRECTION('ref_axis',(-0.809016994374936,0.,-0.587785252292488));
#34881=DIRECTION('',(-0.809016994374936,0.,-0.587785252292488));
#34882=DIRECTION('',(0.,1.,0.));
#34883=DIRECTION('',(-0.809016994374936,0.,-0.587785252292488));
#34884=DIRECTION('',(0.,1.,0.));
#34885=DIRECTION('center_axis',(0.809016994374974,0.,0.587785252292436));
#34886=DIRECTION('ref_axis',(0.587785252292436,0.,-0.809016994374974));
#34887=DIRECTION('',(0.587785252292436,0.,-0.809016994374974));
#34888=DIRECTION('',(0.,1.,0.));
#34889=DIRECTION('',(0.587785252292436,0.,-0.809016994374974));
#34890=DIRECTION('center_axis',(-0.587785252292486,0.,0.809016994374938));
#34891=DIRECTION('ref_axis',(0.809016994374938,0.,0.587785252292486));
#34892=DIRECTION('',(0.809016994374938,0.,0.587785252292486));
#34893=DIRECTION('',(0.,1.,0.));
#34894=DIRECTION('',(0.809016994374938,0.,0.587785252292486));
#34895=DIRECTION('center_axis',(-0.809016994374967,0.,-0.587785252292446));
#34896=DIRECTION('ref_axis',(-0.587785252292446,0.,0.809016994374967));
#34897=DIRECTION('',(-0.587785252292446,0.,0.809016994374967));
#34898=DIRECTION('',(-0.587785252292446,0.,0.809016994374967));
#34899=DIRECTION('center_axis',(0.,1.,0.));
#34900=DIRECTION('ref_axis',(0.,0.,1.));
#34901=DIRECTION('center_axis',(-0.707106781186552,0.,0.707106781186543));
#34902=DIRECTION('ref_axis',(0.707106781186543,0.,0.707106781186552));
#34903=DIRECTION('',(0.707106781186543,0.,0.707106781186552));
#34904=DIRECTION('',(0.,1.,0.));
#34905=DIRECTION('',(0.707106781186543,0.,0.707106781186552));
#34906=DIRECTION('',(0.,1.,0.));
#34907=DIRECTION('center_axis',(-0.707106781186488,0.,-0.707106781186607));
#34908=DIRECTION('ref_axis',(-0.707106781186607,0.,0.707106781186488));
#34909=DIRECTION('',(-0.707106781186607,0.,0.707106781186488));
#34910=DIRECTION('',(0.,1.,0.));
#34911=DIRECTION('',(-0.707106781186607,0.,0.707106781186488));
#34912=DIRECTION('center_axis',(0.707106781186552,0.,-0.707106781186543));
#34913=DIRECTION('ref_axis',(-0.707106781186543,0.,-0.707106781186552));
#34914=DIRECTION('',(-0.707106781186543,0.,-0.707106781186552));
#34915=DIRECTION('',(0.,1.,0.));
#34916=DIRECTION('',(-0.707106781186543,0.,-0.707106781186552));
#34917=DIRECTION('center_axis',(0.707106781186488,0.,0.707106781186607));
#34918=DIRECTION('ref_axis',(0.707106781186607,0.,-0.707106781186488));
#34919=DIRECTION('',(0.707106781186607,0.,-0.707106781186488));
#34920=DIRECTION('',(0.707106781186607,0.,-0.707106781186488));
#34921=DIRECTION('center_axis',(0.,1.,0.));
#34922=DIRECTION('ref_axis',(0.,0.,1.));
#34923=DIRECTION('center_axis',(0.891006524188366,0.,0.45399049973955));
#34924=DIRECTION('ref_axis',(0.45399049973955,0.,-0.891006524188366));
#34925=DIRECTION('',(0.45399049973955,0.,-0.891006524188366));
#34926=DIRECTION('',(0.,1.,0.));
#34927=DIRECTION('',(0.45399049973955,0.,-0.891006524188366));
#34928=DIRECTION('',(0.,1.,0.));
#34929=DIRECTION('center_axis',(-0.453990499739501,0.,0.891006524188391));
#34930=DIRECTION('ref_axis',(0.891006524188391,0.,0.453990499739501));
#34931=DIRECTION('',(0.891006524188391,0.,0.453990499739501));
#34932=DIRECTION('',(0.,1.,0.));
#34933=DIRECTION('',(0.891006524188391,0.,0.453990499739501));
#34934=DIRECTION('center_axis',(-0.891006524188366,0.,-0.45399049973955));
#34935=DIRECTION('ref_axis',(-0.45399049973955,0.,0.891006524188366));
#34936=DIRECTION('',(-0.45399049973955,0.,0.891006524188366));
#34937=DIRECTION('',(0.,1.,0.));
#34938=DIRECTION('',(-0.45399049973955,0.,0.891006524188366));
#34939=DIRECTION('center_axis',(0.453990499739501,0.,-0.891006524188391));
#34940=DIRECTION('ref_axis',(-0.891006524188391,0.,-0.453990499739501));
#34941=DIRECTION('',(-0.891006524188391,0.,-0.453990499739501));
#34942=DIRECTION('',(-0.891006524188391,0.,-0.453990499739501));
#34943=DIRECTION('center_axis',(0.,1.,0.));
#34944=DIRECTION('ref_axis',(0.,0.,1.));
#34945=DIRECTION('center_axis',(0.156434465040221,0.,0.987688340595139));
#34946=DIRECTION('ref_axis',(0.987688340595139,0.,-0.156434465040221));
#34947=DIRECTION('',(0.987688340595139,0.,-0.156434465040221));
#34948=DIRECTION('',(0.,1.,0.));
#34949=DIRECTION('',(0.987688340595139,0.,-0.156434465040221));
#34950=DIRECTION('',(0.,1.,0.));
#34951=DIRECTION('center_axis',(-0.987688340595144,0.,0.156434465040192));
#34952=DIRECTION('ref_axis',(0.156434465040192,0.,0.987688340595144));
#34953=DIRECTION('',(0.156434465040192,0.,0.987688340595144));
#34954=DIRECTION('',(0.,1.,0.));
#34955=DIRECTION('',(0.156434465040192,0.,0.987688340595144));
#34956=DIRECTION('center_axis',(-0.156434465040198,0.,-0.987688340595143));
#34957=DIRECTION('ref_axis',(-0.987688340595143,0.,0.156434465040198));
#34958=DIRECTION('',(-0.987688340595143,0.,0.156434465040198));
#34959=DIRECTION('',(0.,1.,0.));
#34960=DIRECTION('',(-0.987688340595143,0.,0.156434465040198));
#34961=DIRECTION('center_axis',(0.987688340595141,0.,-0.15643446504021));
#34962=DIRECTION('ref_axis',(-0.15643446504021,0.,-0.987688340595141));
#34963=DIRECTION('',(-0.15643446504021,0.,-0.987688340595141));
#34964=DIRECTION('',(-0.15643446504021,0.,-0.987688340595141));
#34965=DIRECTION('center_axis',(0.,1.,0.));
#34966=DIRECTION('ref_axis',(0.,0.,1.));
#34967=DIRECTION('center_axis',(-0.309016994374931,0.,0.951056516295159));
#34968=DIRECTION('ref_axis',(0.951056516295159,0.,0.309016994374931));
#34969=DIRECTION('',(0.951056516295159,0.,0.309016994374931));
#34970=DIRECTION('',(0.,1.,0.));
#34971=DIRECTION('',(0.951056516295159,0.,0.309016994374931));
#34972=DIRECTION('',(0.,1.,0.));
#34973=DIRECTION('center_axis',(-0.951056516295164,0.,-0.309016994374916));
#34974=DIRECTION('ref_axis',(-0.309016994374916,0.,0.951056516295164));
#34975=DIRECTION('',(-0.309016994374916,0.,0.951056516295164));
#34976=DIRECTION('',(0.,1.,0.));
#34977=DIRECTION('',(-0.309016994374916,0.,0.951056516295164));
#34978=DIRECTION('center_axis',(0.309016994374968,0.,-0.951056516295147));
#34979=DIRECTION('ref_axis',(-0.951056516295147,0.,-0.309016994374968));
#34980=DIRECTION('',(-0.951056516295147,0.,-0.309016994374968));
#34981=DIRECTION('',(0.,1.,0.));
#34982=DIRECTION('',(-0.951056516295147,0.,-0.309016994374968));
#34983=DIRECTION('center_axis',(0.951056516295153,0.,0.309016994374951));
#34984=DIRECTION('ref_axis',(0.309016994374951,0.,-0.951056516295153));
#34985=DIRECTION('',(0.309016994374951,0.,-0.951056516295153));
#34986=DIRECTION('',(0.309016994374951,0.,-0.951056516295153));
#34987=DIRECTION('center_axis',(0.,1.,0.));
#34988=DIRECTION('ref_axis',(0.,0.,1.));
#34989=DIRECTION('center_axis',(0.587785252292488,0.,0.809016994374936));
#34990=DIRECTION('ref_axis',(0.809016994374936,0.,-0.587785252292488));
#34991=DIRECTION('',(0.809016994374936,0.,-0.587785252292488));
#34992=DIRECTION('',(0.,1.,0.));
#34993=DIRECTION('',(0.809016994374936,0.,-0.587785252292488));
#34994=DIRECTION('',(0.,1.,0.));
#34995=DIRECTION('center_axis',(-0.809016994374971,0.,0.587785252292441));
#34996=DIRECTION('ref_axis',(0.587785252292441,0.,0.809016994374971));
#34997=DIRECTION('',(0.587785252292441,0.,0.809016994374971));
#34998=DIRECTION('',(0.,1.,0.));
#34999=DIRECTION('',(0.587785252292441,0.,0.809016994374971));
#35000=DIRECTION('center_axis',(-0.587785252292491,0.,-0.809016994374935));
#35001=DIRECTION('ref_axis',(-0.809016994374935,0.,0.587785252292491));
#35002=DIRECTION('',(-0.809016994374935,0.,0.587785252292491));
#35003=DIRECTION('',(0.,1.,0.));
#35004=DIRECTION('',(-0.809016994374935,0.,0.587785252292491));
#35005=DIRECTION('center_axis',(0.809016994374964,0.,-0.587785252292451));
#35006=DIRECTION('ref_axis',(-0.587785252292451,0.,-0.809016994374964));
#35007=DIRECTION('',(-0.587785252292451,0.,-0.809016994374964));
#35008=DIRECTION('',(-0.587785252292451,0.,-0.809016994374964));
#35009=DIRECTION('center_axis',(0.,1.,0.));
#35010=DIRECTION('ref_axis',(0.,0.,1.));
#35011=DIRECTION('center_axis',(1.,0.,0.));
#35012=DIRECTION('ref_axis',(0.,0.,-1.));
#35013=DIRECTION('',(0.,0.,-1.));
#35014=DIRECTION('',(0.,1.,0.));
#35015=DIRECTION('',(0.,0.,-1.));
#35016=DIRECTION('',(0.,1.,0.));
#35017=DIRECTION('center_axis',(0.,0.,1.));
#35018=DIRECTION('ref_axis',(1.,0.,0.));
#35019=DIRECTION('',(1.,0.,0.));
#35020=DIRECTION('',(0.,1.,0.));
#35021=DIRECTION('',(1.,0.,0.));
#35022=DIRECTION('center_axis',(-1.,0.,0.));
#35023=DIRECTION('ref_axis',(0.,0.,1.));
#35024=DIRECTION('',(0.,0.,1.));
#35025=DIRECTION('',(0.,1.,0.));
#35026=DIRECTION('',(0.,0.,1.));
#35027=DIRECTION('center_axis',(0.,0.,-1.));
#35028=DIRECTION('ref_axis',(-1.,0.,0.));
#35029=DIRECTION('',(-1.,0.,0.));
#35030=DIRECTION('',(-1.,0.,0.));
#35031=DIRECTION('center_axis',(0.,1.,0.));
#35032=DIRECTION('ref_axis',(0.,0.,1.));
#35033=DIRECTION('center_axis',(0.891006524188366,0.,-0.453990499739551));
#35034=DIRECTION('ref_axis',(-0.453990499739551,0.,-0.891006524188366));
#35035=DIRECTION('',(-0.453990499739551,0.,-0.891006524188366));
#35036=DIRECTION('',(0.,1.,0.));
#35037=DIRECTION('',(-0.453990499739551,0.,-0.891006524188366));
#35038=DIRECTION('',(0.,1.,0.));
#35039=DIRECTION('center_axis',(0.453990499739501,0.,0.891006524188391));
#35040=DIRECTION('ref_axis',(0.891006524188391,0.,-0.453990499739501));
#35041=DIRECTION('',(0.891006524188391,0.,-0.453990499739501));
#35042=DIRECTION('',(0.,1.,0.));
#35043=DIRECTION('',(0.891006524188391,0.,-0.453990499739501));
#35044=DIRECTION('center_axis',(-0.891006524188366,0.,0.453990499739551));
#35045=DIRECTION('ref_axis',(0.453990499739551,0.,0.891006524188366));
#35046=DIRECTION('',(0.453990499739551,0.,0.891006524188366));
#35047=DIRECTION('',(0.,1.,0.));
#35048=DIRECTION('',(0.453990499739551,0.,0.891006524188366));
#35049=DIRECTION('center_axis',(-0.453990499739501,0.,-0.891006524188391));
#35050=DIRECTION('ref_axis',(-0.891006524188391,0.,0.453990499739501));
#35051=DIRECTION('',(-0.891006524188391,0.,0.453990499739501));
#35052=DIRECTION('',(-0.891006524188391,0.,0.453990499739501));
#35053=DIRECTION('center_axis',(0.,1.,0.));
#35054=DIRECTION('ref_axis',(0.,0.,1.));
#35055=DIRECTION('center_axis',(0.156434465040197,0.,-0.987688340595143));
#35056=DIRECTION('ref_axis',(-0.987688340595143,0.,-0.156434465040197));
#35057=DIRECTION('',(-0.987688340595143,0.,-0.156434465040197));
#35058=DIRECTION('',(0.,1.,0.));
#35059=DIRECTION('',(-0.987688340595143,0.,-0.156434465040197));
#35060=DIRECTION('',(0.,1.,0.));
#35061=DIRECTION('center_axis',(0.987688340595143,0.,0.156434465040199));
#35062=DIRECTION('ref_axis',(0.156434465040199,0.,-0.987688340595143));
#35063=DIRECTION('',(0.156434465040199,0.,-0.987688340595143));
#35064=DIRECTION('',(0.,1.,0.));
#35065=DIRECTION('',(0.156434465040199,0.,-0.987688340595143));
#35066=DIRECTION('center_axis',(-0.156434465040221,0.,0.987688340595139));
#35067=DIRECTION('ref_axis',(0.987688340595139,0.,0.156434465040221));
#35068=DIRECTION('',(0.987688340595139,0.,0.156434465040221));
#35069=DIRECTION('',(0.,1.,0.));
#35070=DIRECTION('',(0.987688340595139,0.,0.156434465040221));
#35071=DIRECTION('center_axis',(-0.987688340595141,0.,-0.15643446504021));
#35072=DIRECTION('ref_axis',(-0.15643446504021,0.,0.987688340595141));
#35073=DIRECTION('',(-0.15643446504021,0.,0.987688340595141));
#35074=DIRECTION('',(-0.15643446504021,0.,0.987688340595141));
#35075=DIRECTION('center_axis',(0.,1.,0.));
#35076=DIRECTION('ref_axis',(0.,0.,1.));
#35077=DIRECTION('center_axis',(-0.707106781186553,0.,-0.707106781186542));
#35078=DIRECTION('ref_axis',(-0.707106781186542,0.,0.707106781186553));
#35079=DIRECTION('',(-0.707106781186542,0.,0.707106781186553));
#35080=DIRECTION('',(0.,1.,0.));
#35081=DIRECTION('',(-0.707106781186542,0.,0.707106781186553));
#35082=DIRECTION('',(0.,1.,0.));
#35083=DIRECTION('center_axis',(0.707106781186488,0.,-0.707106781186607));
#35084=DIRECTION('ref_axis',(-0.707106781186607,0.,-0.707106781186488));
#35085=DIRECTION('',(-0.707106781186607,0.,-0.707106781186488));
#35086=DIRECTION('',(0.,1.,0.));
#35087=DIRECTION('',(-0.707106781186607,0.,-0.707106781186488));
#35088=DIRECTION('center_axis',(0.707106781186553,0.,0.707106781186542));
#35089=DIRECTION('ref_axis',(0.707106781186542,0.,-0.707106781186553));
#35090=DIRECTION('',(0.707106781186542,0.,-0.707106781186553));
#35091=DIRECTION('',(0.,1.,0.));
#35092=DIRECTION('',(0.707106781186542,0.,-0.707106781186553));
#35093=DIRECTION('center_axis',(-0.707106781186488,0.,0.707106781186607));
#35094=DIRECTION('ref_axis',(0.707106781186607,0.,0.707106781186488));
#35095=DIRECTION('',(0.707106781186607,0.,0.707106781186488));
#35096=DIRECTION('',(0.707106781186607,0.,0.707106781186488));
#35097=DIRECTION('center_axis',(0.,1.,0.));
#35098=DIRECTION('ref_axis',(0.,0.,1.));
#35099=DIRECTION('center_axis',(0.,1.,0.));
#35100=DIRECTION('ref_axis',(0.,0.,1.));
#35101=DIRECTION('center_axis',(0.,-1.,0.));
#35102=DIRECTION('ref_axis',(1.,0.,0.));
#35103=DIRECTION('center_axis',(0.,-1.,0.));
#35104=DIRECTION('ref_axis',(1.,0.,0.));
#35105=DIRECTION('',(0.,-1.,0.));
#35106=DIRECTION('center_axis',(0.,1.,0.));
#35107=DIRECTION('ref_axis',(1.,0.,0.));
#35108=DIRECTION('center_axis',(0.,1.,0.));
#35109=DIRECTION('ref_axis',(0.,0.,1.));
#35110=DIRECTION('center_axis',(0.,-1.,0.));
#35111=DIRECTION('ref_axis',(1.,0.,0.));
#35112=DIRECTION('center_axis',(0.,-1.,0.));
#35113=DIRECTION('ref_axis',(1.,0.,0.));
#35114=DIRECTION('center_axis',(0.,-1.,0.));
#35115=DIRECTION('ref_axis',(1.,0.,0.));
#35116=DIRECTION('',(0.707106781186548,0.707106781186547,8.65956056235494E-17));
#35117=DIRECTION('center_axis',(0.,-1.,0.));
#35118=DIRECTION('ref_axis',(1.,0.,0.));
#35119=DIRECTION('center_axis',(0.,-1.,0.));
#35120=DIRECTION('ref_axis',(1.,0.,0.));
#35121=DIRECTION('',(0.,1.,0.));
#35122=DIRECTION('center_axis',(0.,1.,0.));
#35123=DIRECTION('ref_axis',(0.,0.,1.));
#35124=DIRECTION('center_axis',(0.,-1.,0.));
#35125=DIRECTION('ref_axis',(1.,0.,0.));
#35126=DIRECTION('center_axis',(0.,-1.,0.));
#35127=DIRECTION('ref_axis',(1.,0.,0.));
#35128=DIRECTION('center_axis',(0.,-1.,0.));
#35129=DIRECTION('ref_axis',(1.,0.,0.));
#35130=DIRECTION('',(0.,1.,0.));
#35131=DIRECTION('center_axis',(0.,1.,0.));
#35132=DIRECTION('ref_axis',(1.,0.,0.));
#35133=DIRECTION('center_axis',(0.,-1.,0.));
#35134=DIRECTION('ref_axis',(1.,0.,0.));
#35135=DIRECTION('',(-0.707106781186547,0.707106781186548,-8.65956056235492E-17));
#35136=DIRECTION('center_axis',(0.,-1.,0.));
#35137=DIRECTION('ref_axis',(0.,0.,-1.));
#48688=CARTESIAN_POINT('',(0.,0.,0.));
#48689=CARTESIAN_POINT('Origin',(-8.5,0.,109.7));
#48690=CARTESIAN_POINT('',(-8.9,-4.89858719658942E-17,112.75));
#48691=CARTESIAN_POINT('Origin',(-8.5,0.,112.75));
#48692=CARTESIAN_POINT('',(-8.9,-4.89858719658942E-17,109.7));
#48693=CARTESIAN_POINT('',(-8.9,-4.89858719658942E-17,109.7));
#48694=CARTESIAN_POINT('Origin',(-8.5,0.,109.7));
#48695=CARTESIAN_POINT('Origin',(-8.5,0.,109.7));
#48696=CARTESIAN_POINT('Origin',(-8.5,0.,113.95));
#48697=CARTESIAN_POINT('',(-8.09585481156726,-0.7,113.95));
#48698=CARTESIAN_POINT('',(-7.69170962313452,0.,113.95));
#48699=CARTESIAN_POINT('',(-8.09585481156726,-0.7,113.95));
#48700=CARTESIAN_POINT('',(-8.09585481156726,0.7,113.95));
#48701=CARTESIAN_POINT('',(-7.69170962313452,0.,113.95));
#48702=CARTESIAN_POINT('',(-8.90414518843274,0.7,113.95));
#48703=CARTESIAN_POINT('',(-8.09585481156726,0.7,113.95));
#48704=CARTESIAN_POINT('',(-9.30829037686548,1.11022302462516E-16,113.95));
#48705=CARTESIAN_POINT('',(-8.90414518843274,0.7,113.95));
#48706=CARTESIAN_POINT('',(-8.90414518843274,-0.7,113.95));
#48707=CARTESIAN_POINT('',(-9.30829037686548,9.89870222809913E-17,113.95));
#48708=CARTESIAN_POINT('',(-8.90414518843274,-0.7,113.95));
#48709=CARTESIAN_POINT('',(-9.1,-7.34788079488412E-17,113.95));
#48710=CARTESIAN_POINT('Origin',(-8.5,0.,113.95));
#48711=CARTESIAN_POINT('Origin',(-8.90414518843274,-0.7,112.75));
#48712=CARTESIAN_POINT('',(-8.90414518843274,-0.7,112.75));
#48713=CARTESIAN_POINT('',(-8.09585481156726,-0.7,112.75));
#48714=CARTESIAN_POINT('',(-8.90414518843274,-0.7,112.75));
#48715=CARTESIAN_POINT('',(-8.09585481156726,-0.7,112.75));
#48716=CARTESIAN_POINT('',(-8.90414518843274,-0.7,112.75));
#48717=CARTESIAN_POINT('Origin',(-9.30829037686548,9.89870222809913E-17,
112.75));
#48718=CARTESIAN_POINT('',(-9.30829037686548,9.89870222809913E-17,112.75));
#48719=CARTESIAN_POINT('',(-9.30829037686548,9.89870222809913E-17,112.75));
#48720=CARTESIAN_POINT('',(-9.30829037686548,9.89870222809913E-17,112.75));
#48721=CARTESIAN_POINT('Origin',(-8.90414518843274,0.7,112.75));
#48722=CARTESIAN_POINT('',(-8.90414518843274,0.7,112.75));
#48723=CARTESIAN_POINT('',(-8.90414518843274,0.7,112.75));
#48724=CARTESIAN_POINT('',(-8.90414518843274,0.7,112.75));
#48725=CARTESIAN_POINT('Origin',(-8.09585481156726,0.7,112.75));
#48726=CARTESIAN_POINT('',(-8.09585481156726,0.7,112.75));
#48727=CARTESIAN_POINT('',(-8.09585481156726,0.7,112.75));
#48728=CARTESIAN_POINT('',(-8.09585481156726,0.7,112.75));
#48729=CARTESIAN_POINT('Origin',(-7.69170962313452,0.,112.75));
#48730=CARTESIAN_POINT('',(-7.69170962313452,0.,112.75));
#48731=CARTESIAN_POINT('',(-7.69170962313452,0.,112.75));
#48732=CARTESIAN_POINT('',(-7.69170962313452,0.,112.75));
#48733=CARTESIAN_POINT('Origin',(-8.09585481156726,-0.7,112.75));
#48734=CARTESIAN_POINT('',(-8.09585481156726,-0.7,112.75));
#48735=CARTESIAN_POINT('Origin',(-8.5,0.,112.75));
#48736=CARTESIAN_POINT('Origin',(-8.5,0.,115.4));
#48737=CARTESIAN_POINT('',(-7.94098300562502,-0.217944947176943,115.4));
#48738=CARTESIAN_POINT('',(-7.94098300562502,0.217944947176943,115.4));
#48739=CARTESIAN_POINT('',(-7.94098300562502,0.,115.4));
#48740=CARTESIAN_POINT('Origin',(-8.5,0.,115.4));
#48741=CARTESIAN_POINT('Origin',(-8.5,0.,115.4));
#48742=CARTESIAN_POINT('',(-9.05901699437498,0.217944947176943,115.4));
#48743=CARTESIAN_POINT('',(-9.05901699437498,-0.217944947176943,115.4));
#48744=CARTESIAN_POINT('',(-9.05901699437498,0.,115.4));
#48745=CARTESIAN_POINT('',(-9.1,-7.34788079488412E-17,115.4));
#48746=CARTESIAN_POINT('Origin',(-8.5,0.,115.4));
#48747=CARTESIAN_POINT('Origin',(-8.5,0.,115.4));
#48748=CARTESIAN_POINT('Origin',(-8.5,0.,113.95));
#48749=CARTESIAN_POINT('Ctrl Pts',(-9.05901699437498,-0.217944947176941,
115.4));
#48750=CARTESIAN_POINT('Ctrl Pts',(-9.05746114535787,-0.221935615703616,
115.399719436761));
#48751=CARTESIAN_POINT('Ctrl Pts',(-9.05586245181257,-0.225909893277269,
115.399432356204));
#48752=CARTESIAN_POINT('Ctrl Pts',(-9.02357718014127,-0.303751656945718,
115.393661962552));
#48753=CARTESIAN_POINT('Ctrl Pts',(-8.97743240350865,-0.371095733915202,
115.385929127254));
#48754=CARTESIAN_POINT('Ctrl Pts',(-8.87109817623925,-0.477429961184608,
115.371475590715));
#48755=CARTESIAN_POINT('Ctrl Pts',(-8.80375305869836,-0.523576651819584,
115.363804435153));
#48756=CARTESIAN_POINT('Ctrl Pts',(-8.65597871120912,-0.584866716033612,
115.352992026863));
#48757=CARTESIAN_POINT('Ctrl Pts',(-8.57553441616499,-0.6,115.35));
#48758=CARTESIAN_POINT('Ctrl Pts',(-8.42446558383501,-0.6,115.35));
#48759=CARTESIAN_POINT('Ctrl Pts',(-8.34402128879088,-0.584866716033612,
115.352992026863));
#48760=CARTESIAN_POINT('Ctrl Pts',(-8.19624694130164,-0.523576651819584,
115.363804435153));
#48761=CARTESIAN_POINT('Ctrl Pts',(-8.12890182376075,-0.477429961184608,
115.371475590715));
#48762=CARTESIAN_POINT('Ctrl Pts',(-8.02256759649135,-0.371095733915202,
115.385929127254));
#48763=CARTESIAN_POINT('Ctrl Pts',(-7.97642281985873,-0.303751656945718,
115.393661962552));
#48764=CARTESIAN_POINT('Ctrl Pts',(-7.94413754818743,-0.225909893277269,
115.399432356204));
#48765=CARTESIAN_POINT('Ctrl Pts',(-7.94253885464213,-0.221935615703617,
115.399719436761));
#48766=CARTESIAN_POINT('Ctrl Pts',(-7.94098300562502,-0.217944947176942,
115.4));
#48767=CARTESIAN_POINT('',(-9.1,-7.34788079488412E-17,113.95));
#48768=CARTESIAN_POINT('Ctrl Pts',(-7.94098300562502,0.217944947176942,
115.4));
#48769=CARTESIAN_POINT('Ctrl Pts',(-7.94253885464213,0.221935615703616,
115.399719436761));
#48770=CARTESIAN_POINT('Ctrl Pts',(-7.94413754818743,0.225909893277269,
115.399432356204));
#48771=CARTESIAN_POINT('Ctrl Pts',(-7.97642281985873,0.303751656945718,
115.393661962552));
#48772=CARTESIAN_POINT('Ctrl Pts',(-8.02256759649135,0.371095733915202,
115.385929127254));
#48773=CARTESIAN_POINT('Ctrl Pts',(-8.12890182376075,0.477429961184608,
115.371475590715));
#48774=CARTESIAN_POINT('Ctrl Pts',(-8.19624694130164,0.523576651819582,
115.363804435153));
#48775=CARTESIAN_POINT('Ctrl Pts',(-8.34402128879088,0.584866716033611,
115.352992026863));
#48776=CARTESIAN_POINT('Ctrl Pts',(-8.42446558383501,0.6,115.35));
#48777=CARTESIAN_POINT('Ctrl Pts',(-8.57553441616499,0.6,115.35));
#48778=CARTESIAN_POINT('Ctrl Pts',(-8.65597871120912,0.584866716033612,
115.352992026863));
#48779=CARTESIAN_POINT('Ctrl Pts',(-8.80375305869836,0.523576651819584,
115.363804435153));
#48780=CARTESIAN_POINT('Ctrl Pts',(-8.87109817623925,0.477429961184608,
115.371475590715));
#48781=CARTESIAN_POINT('Ctrl Pts',(-8.97743240350865,0.371095733915202,
115.385929127254));
#48782=CARTESIAN_POINT('Ctrl Pts',(-9.02357718014127,0.30375165694572,115.393661962552));
#48783=CARTESIAN_POINT('Ctrl Pts',(-9.05586245181257,0.22590989327727,115.399432356204));
#48784=CARTESIAN_POINT('Ctrl Pts',(-9.05746114535787,0.221935615703616,
115.399719436761));
#48785=CARTESIAN_POINT('Ctrl Pts',(-9.05901699437498,0.217944947176941,
115.4));
#48786=CARTESIAN_POINT('Origin',(-8.5,-1.5,118.5));
#48787=CARTESIAN_POINT('',(-8.68357599741213,-1.5,118.737275900955));
#48788=CARTESIAN_POINT('',(-8.20011630702142,-1.5,118.491647115137));
#48789=CARTESIAN_POINT('Origin',(-8.5,-1.5,118.5));
#48790=CARTESIAN_POINT('',(-8.68357599741213,-1.6,118.737275900955));
#48791=CARTESIAN_POINT('',(-8.68357599741213,-1.5,118.737275900955));
#48792=CARTESIAN_POINT('',(-8.20011630702142,-1.6,118.491647115137));
#48793=CARTESIAN_POINT('Origin',(-8.5,-1.6,118.5));
#48794=CARTESIAN_POINT('',(-8.20011630702142,-1.5,118.491647115137));
#48795=CARTESIAN_POINT('Origin',(-8.07858983848623,-1.5,118.429903810568));
#48796=CARTESIAN_POINT('',(-8.07858983848623,-1.5,118.429903810568));
#48797=CARTESIAN_POINT('',(-7.10771361113469,-1.5,117.936635905003));
#48798=CARTESIAN_POINT('',(-8.07858983848623,-1.6,118.429903810568));
#48799=CARTESIAN_POINT('',(-8.07858983848623,-1.6,118.429903810568));
#48800=CARTESIAN_POINT('',(-8.07858983848623,-1.5,118.429903810568));
#48801=CARTESIAN_POINT('Origin',(-8.22858983848623,-1.5,118.170096189432));
#48802=CARTESIAN_POINT('',(-8.22858983848623,-1.5,118.170096189432));
#48803=CARTESIAN_POINT('',(-7.82858983848618,-1.5,118.86291651246));
#48804=CARTESIAN_POINT('',(-8.22858983848623,-1.6,118.170096189432));
#48805=CARTESIAN_POINT('',(-8.22858983848623,-1.6,118.170096189432));
#48806=CARTESIAN_POINT('',(-8.22858983848623,-1.5,118.170096189432));
#48807=CARTESIAN_POINT('Origin',(-8.34282434302488,-1.5,118.244469546131));
#48808=CARTESIAN_POINT('',(-8.34282434302488,-1.5,118.244469546131));
#48809=CARTESIAN_POINT('',(-7.43809082420648,-1.5,117.655435007187));
#48810=CARTESIAN_POINT('',(-8.34282434302488,-1.6,118.244469546131));
#48811=CARTESIAN_POINT('',(-10.5784609690827,-1.6,119.7));
#48812=CARTESIAN_POINT('',(-8.34282434302488,-1.5,118.244469546131));
#48813=CARTESIAN_POINT('Origin',(-8.5,-1.5,118.5));
#48814=CARTESIAN_POINT('',(-8.79727495663918,-1.5,118.540343526806));
#48815=CARTESIAN_POINT('Origin',(-8.5,-1.5,118.5));
#48816=CARTESIAN_POINT('',(-8.79727495663918,-1.6,118.540343526806));
#48817=CARTESIAN_POINT('Origin',(-8.5,-1.6,118.5));
#48818=CARTESIAN_POINT('',(-8.79727495663918,-1.5,118.540343526806));
#48819=CARTESIAN_POINT('Origin',(-10.5784609690827,-1.5,119.7));
#48820=CARTESIAN_POINT('',(-10.5784609690827,-1.5,119.7));
#48821=CARTESIAN_POINT('',(-8.55590913723536,-1.5,118.383200234122));
#48822=CARTESIAN_POINT('',(-10.5784609690827,-1.6,119.7));
#48823=CARTESIAN_POINT('',(-10.5784609690827,-1.6,119.7));
#48824=CARTESIAN_POINT('',(-10.5784609690827,-1.5,119.7));
#48825=CARTESIAN_POINT('Origin',(-8.68357599741213,-1.5,118.737275900955));
#48826=CARTESIAN_POINT('',(-7.41020669059764,-1.5,118.090321950197));
#48827=CARTESIAN_POINT('',(-8.07858983848623,-1.6,118.429903810568));
#48828=CARTESIAN_POINT('Origin',(-9.32852540378444,-1.6,118.935048094716));
#48829=CARTESIAN_POINT('Origin',(-5.95068842566558,-1.5,117.60859072421));
#48830=CARTESIAN_POINT('',(-5.95068842566558,-1.5,117.60859072421));
#48831=CARTESIAN_POINT('',(-6.28355820636889,-1.5,117.716746672241));
#48832=CARTESIAN_POINT('',(-5.92307740174221,-1.5,117.599619358704));
#48833=CARTESIAN_POINT('',(-5.95068842566558,-1.45,117.60859072421));
#48834=CARTESIAN_POINT('',(-5.95068842566558,-1.5,117.60859072421));
#48835=CARTESIAN_POINT('',(-6.28355820636889,-1.45,117.716746672241));
#48836=CARTESIAN_POINT('',(-5.95068842566558,-1.45,117.60859072421));
#48837=CARTESIAN_POINT('',(-6.28355820636889,-1.5,117.716746672241));
#48838=CARTESIAN_POINT('Origin',(-5.91360638634059,-1.5,117.722717506165));
#48839=CARTESIAN_POINT('',(-5.91360638634059,-1.5,117.722717506165));
#48840=CARTESIAN_POINT('',(-5.78441421709369,-1.5,118.120330118589));
#48841=CARTESIAN_POINT('',(-5.91360638634059,-1.45,117.722717506165));
#48842=CARTESIAN_POINT('',(-5.91360638634059,-1.5,117.722717506165));
#48843=CARTESIAN_POINT('',(-5.91360638634059,-1.45,117.722717506165));
#48844=CARTESIAN_POINT('Origin',(-6.24647616704389,-1.5,117.830873454197));
#48845=CARTESIAN_POINT('',(-6.24647616704389,-1.5,117.830873454197));
#48846=CARTESIAN_POINT('',(-6.05243025276885,-1.5,117.767824114675));
#48847=CARTESIAN_POINT('',(-6.24647616704389,-1.45,117.830873454197));
#48848=CARTESIAN_POINT('',(-6.24647616704389,-1.5,117.830873454197));
#48849=CARTESIAN_POINT('',(-6.24647616704389,-1.45,117.830873454197));
#48850=CARTESIAN_POINT('Origin',(-6.28355820636889,-1.5,117.716746672241));
#48851=CARTESIAN_POINT('',(-6.13582501745948,-1.5,118.171422675642));
#48852=CARTESIAN_POINT('',(-6.28355820636889,-1.45,117.716746672241));
#48853=CARTESIAN_POINT('Origin',(-6.09858229635474,-1.45,117.719732089203));
#48854=CARTESIAN_POINT('Origin',(-6.28038700005009,-1.5,120.038479161527));
#48855=CARTESIAN_POINT('',(-6.28038700005009,-1.5,120.038479161527));
#48856=CARTESIAN_POINT('',(-6.56354294808132,-1.5,119.832754323225));
#48857=CARTESIAN_POINT('',(-6.42352262153444,-1.5,119.934485045246));
#48858=CARTESIAN_POINT('',(-6.28038700005009,-1.45,120.038479161527));
#48859=CARTESIAN_POINT('',(-6.28038700005009,-1.5,120.038479161527));
#48860=CARTESIAN_POINT('',(-6.56354294808132,-1.45,119.832754323225));
#48861=CARTESIAN_POINT('',(-6.28038700005009,-1.45,120.038479161527));
#48862=CARTESIAN_POINT('',(-6.56354294808132,-1.5,119.832754323225));
#48863=CARTESIAN_POINT('Origin',(-6.35092123032519,-1.5,120.135561200852));
#48864=CARTESIAN_POINT('',(-6.35092123032519,-1.5,120.135561200852));
#48865=CARTESIAN_POINT('',(-5.83232499367828,-1.5,119.421774716707));
#48866=CARTESIAN_POINT('',(-6.35092123032519,-1.45,120.135561200852));
#48867=CARTESIAN_POINT('',(-6.35092123032519,-1.5,120.135561200852));
#48868=CARTESIAN_POINT('',(-6.35092123032519,-1.45,120.135561200852));
#48869=CARTESIAN_POINT('Origin',(-6.63407717835642,-1.5,119.92983636255));
#48870=CARTESIAN_POINT('',(-6.63407717835642,-1.5,119.92983636255));
#48871=CARTESIAN_POINT('',(-6.63563482582516,-1.5,119.92870466542));
#48872=CARTESIAN_POINT('',(-6.63407717835642,-1.45,119.92983636255));
#48873=CARTESIAN_POINT('',(-6.63407717835642,-1.5,119.92983636255));
#48874=CARTESIAN_POINT('',(-6.63407717835642,-1.45,119.92983636255));
#48875=CARTESIAN_POINT('Origin',(-6.56354294808132,-1.5,119.832754323225));
#48876=CARTESIAN_POINT('',(-6.08021382657196,-1.5,119.167508858742));
#48877=CARTESIAN_POINT('',(-6.56354294808132,-1.45,119.832754323225));
#48878=CARTESIAN_POINT('Origin',(-6.45723208920326,-1.45,119.984157762038));
#48879=CARTESIAN_POINT('Origin',(-10.4516147160749,-1.5,116.633238097668));
#48880=CARTESIAN_POINT('',(-10.4516147160749,-1.5,116.633238097668));
#48881=CARTESIAN_POINT('',(-10.0273506473629,-1.5,117.057502166379));
#48882=CARTESIAN_POINT('',(-8.77202056147305,-1.5,118.312832252269));
#48883=CARTESIAN_POINT('',(-10.4516147160749,-1.45,116.633238097668));
#48884=CARTESIAN_POINT('',(-10.4516147160749,-1.5,116.633238097668));
#48885=CARTESIAN_POINT('',(-10.0273506473629,-1.45,117.057502166379));
#48886=CARTESIAN_POINT('',(-10.4516147160749,-1.45,116.633238097668));
#48887=CARTESIAN_POINT('',(-10.0273506473629,-1.5,117.057502166379));
#48888=CARTESIAN_POINT('Origin',(-10.3667619023325,-1.5,116.548385283925));
#48889=CARTESIAN_POINT('',(-10.3667619023325,-1.5,116.548385283925));
#48890=CARTESIAN_POINT('',(-9.66297510576788,-1.5,115.844598487361));
#48891=CARTESIAN_POINT('',(-10.3667619023325,-1.45,116.548385283925));
#48892=CARTESIAN_POINT('',(-10.3667619023325,-1.5,116.548385283925));
#48893=CARTESIAN_POINT('',(-10.3667619023325,-1.45,116.548385283925));
#48894=CARTESIAN_POINT('Origin',(-9.94249783362056,-1.5,116.972649352637));
#48895=CARTESIAN_POINT('',(-9.94249783362056,-1.5,116.972649352637));
#48896=CARTESIAN_POINT('',(-8.4750357133747,-1.5,118.440111472883));
#48897=CARTESIAN_POINT('',(-9.94249783362056,-1.45,116.972649352637));
#48898=CARTESIAN_POINT('',(-9.94249783362056,-1.5,116.972649352637));
#48899=CARTESIAN_POINT('',(-9.94249783362056,-1.45,116.972649352637));
#48900=CARTESIAN_POINT('Origin',(-10.0273506473629,-1.5,117.057502166379));
#48901=CARTESIAN_POINT('',(-9.28113744392716,-1.5,116.311288962944));
#48902=CARTESIAN_POINT('',(-10.0273506473629,-1.45,117.057502166379));
#48903=CARTESIAN_POINT('Origin',(-10.1970562748477,-1.45,116.802943725152));
#48904=CARTESIAN_POINT('Origin',(-9.67231395784547,-1.5,120.932957045293));
#48905=CARTESIAN_POINT('',(-9.67231395784547,-1.5,120.932957045293));
#48906=CARTESIAN_POINT('',(-9.39991965800175,-1.5,120.39835313078));
#48907=CARTESIAN_POINT('',(-8.76057109110912,-1.5,119.143560916717));
#48908=CARTESIAN_POINT('',(-9.67231395784547,-1.45,120.932957045293));
#48909=CARTESIAN_POINT('',(-9.67231395784547,-1.5,120.932957045293));
#48910=CARTESIAN_POINT('',(-9.39991965800175,-1.45,120.39835313078));
#48911=CARTESIAN_POINT('',(-9.67231395784547,-1.45,120.932957045293));
#48912=CARTESIAN_POINT('',(-9.39991965800175,-1.5,120.39835313078));
#48913=CARTESIAN_POINT('Origin',(-9.77923474074808,-1.5,120.878478185324));
#48914=CARTESIAN_POINT('',(-9.77923474074808,-1.5,120.878478185324));
#48915=CARTESIAN_POINT('',(-8.60136023711026,-1.5,121.478635221238));
#48916=CARTESIAN_POINT('',(-9.77923474074808,-1.45,120.878478185324));
#48917=CARTESIAN_POINT('',(-9.77923474074808,-1.5,120.878478185324));
#48918=CARTESIAN_POINT('',(-9.77923474074808,-1.45,120.878478185324));
#48919=CARTESIAN_POINT('Origin',(-9.50684044090435,-1.5,120.343874270811));
#48920=CARTESIAN_POINT('',(-9.50684044090435,-1.5,120.343874270811));
#48921=CARTESIAN_POINT('',(-8.73129472408986,-1.5,118.821780099492));
#48922=CARTESIAN_POINT('',(-9.50684044090435,-1.45,120.343874270811));
#48923=CARTESIAN_POINT('',(-9.50684044090435,-1.5,120.343874270811));
#48924=CARTESIAN_POINT('',(-9.50684044090435,-1.45,120.343874270811));
#48925=CARTESIAN_POINT('Origin',(-9.39991965800175,-1.5,120.39835313078));
#48926=CARTESIAN_POINT('',(-8.27550554581525,-1.5,120.97127073671));
#48927=CARTESIAN_POINT('',(-9.39991965800175,-1.45,120.39835313078));
#48928=CARTESIAN_POINT('Origin',(-9.58957719937491,-1.45,120.638415658052));
#48929=CARTESIAN_POINT('Origin',(-11.1573724517045,-1.5,118.981634356044));
#48930=CARTESIAN_POINT('',(-11.1573724517045,-1.5,118.981634356044));
#48931=CARTESIAN_POINT('',(-10.5647594473474,-1.5,118.88777367702));
#48932=CARTESIAN_POINT('',(-8.40947721758703,-1.5,118.546410507318));
#48933=CARTESIAN_POINT('',(-11.1573724517045,-1.45,118.981634356044));
#48934=CARTESIAN_POINT('',(-11.1573724517045,-1.5,118.981634356044));
#48935=CARTESIAN_POINT('',(-10.5647594473474,-1.45,118.88777367702));
#48936=CARTESIAN_POINT('',(-11.1573724517045,-1.45,118.981634356044));
#48937=CARTESIAN_POINT('',(-10.5647594473474,-1.5,118.88777367702));
#48938=CARTESIAN_POINT('Origin',(-11.1761445875093,-1.5,118.863111755173));
#48939=CARTESIAN_POINT('',(-11.1761445875093,-1.5,118.863111755173));
#48940=CARTESIAN_POINT('',(-11.1359675278721,-1.5,119.116779726312));
#48941=CARTESIAN_POINT('',(-11.1761445875093,-1.45,118.863111755173));
#48942=CARTESIAN_POINT('',(-11.1761445875093,-1.5,118.863111755173));
#48943=CARTESIAN_POINT('',(-11.1761445875093,-1.45,118.863111755173));
#48944=CARTESIAN_POINT('Origin',(-10.5835315831522,-1.5,118.769251076149));
#48945=CARTESIAN_POINT('',(-10.5835315831522,-1.5,118.769251076149));
#48946=CARTESIAN_POINT('',(-8.1319428512133,-1.5,118.380957566935));
#48947=CARTESIAN_POINT('',(-10.5835315831522,-1.45,118.769251076149));
#48948=CARTESIAN_POINT('',(-10.5835315831522,-1.5,118.769251076149));
#48949=CARTESIAN_POINT('',(-10.5835315831522,-1.45,118.769251076149));
#48950=CARTESIAN_POINT('Origin',(-10.5647594473474,-1.5,118.88777367702));
#48951=CARTESIAN_POINT('',(-10.5339684556126,-1.5,119.082180347724));
#48952=CARTESIAN_POINT('',(-10.5647594473474,-1.45,118.88777367702));
#48953=CARTESIAN_POINT('Origin',(-10.8704520174283,-1.45,118.875442716097));
#48954=CARTESIAN_POINT('Origin',(-11.0863936136594,-1.5,117.722717506165));
#48955=CARTESIAN_POINT('',(-11.0863936136594,-1.5,117.722717506165));
#48956=CARTESIAN_POINT('',(-10.7535238329561,-1.5,117.830873454197));
#48957=CARTESIAN_POINT('',(-8.4909299957391,-1.5,118.566034756484));
#48958=CARTESIAN_POINT('',(-11.0863936136594,-1.45,117.722717506165));
#48959=CARTESIAN_POINT('',(-11.0863936136594,-1.5,117.722717506165));
#48960=CARTESIAN_POINT('',(-10.7535238329561,-1.45,117.830873454197));
#48961=CARTESIAN_POINT('',(-11.0863936136594,-1.45,117.722717506165));
#48962=CARTESIAN_POINT('',(-10.7535238329561,-1.5,117.830873454197));
#48963=CARTESIAN_POINT('Origin',(-11.0493115743344,-1.5,117.60859072421));
#48964=CARTESIAN_POINT('',(-11.0493115743344,-1.5,117.60859072421));
#48965=CARTESIAN_POINT('',(-10.9201194050875,-1.5,117.210978111787));
#48966=CARTESIAN_POINT('',(-11.0493115743344,-1.45,117.60859072421));
#48967=CARTESIAN_POINT('',(-11.0493115743344,-1.5,117.60859072421));
#48968=CARTESIAN_POINT('',(-11.0493115743344,-1.45,117.60859072421));
#48969=CARTESIAN_POINT('Origin',(-10.7164417936311,-1.5,117.716746672241));
#48970=CARTESIAN_POINT('',(-10.7164417936311,-1.5,117.716746672241));
#48971=CARTESIAN_POINT('',(-8.2874130660625,-1.5,118.505985948544));
#48972=CARTESIAN_POINT('',(-10.7164417936311,-1.45,117.716746672241));
#48973=CARTESIAN_POINT('',(-10.7164417936311,-1.5,117.716746672241));
#48974=CARTESIAN_POINT('',(-10.7164417936311,-1.45,117.716746672241));
#48975=CARTESIAN_POINT('Origin',(-10.7535238329561,-1.5,117.830873454197));
#48976=CARTESIAN_POINT('',(-10.6057906440467,-1.5,117.376197450796));
#48977=CARTESIAN_POINT('',(-10.7535238329561,-1.45,117.830873454197));
#48978=CARTESIAN_POINT('Origin',(-10.9014177036453,-1.45,117.719732089203));
#48979=CARTESIAN_POINT('Origin',(-10.6490787696748,-1.5,120.135561200852));
#48980=CARTESIAN_POINT('',(-10.6490787696748,-1.5,120.135561200852));
#48981=CARTESIAN_POINT('',(-10.3659228216436,-1.5,119.92983636255));
#48982=CARTESIAN_POINT('',(-8.60786850634683,-1.5,118.652535135943));
#48983=CARTESIAN_POINT('',(-10.6490787696748,-1.45,120.135561200852));
#48984=CARTESIAN_POINT('',(-10.6490787696748,-1.5,120.135561200852));
#48985=CARTESIAN_POINT('',(-10.3659228216436,-1.45,119.92983636255));
#48986=CARTESIAN_POINT('',(-10.6490787696748,-1.45,120.135561200852));
#48987=CARTESIAN_POINT('',(-10.3659228216436,-1.5,119.92983636255));
#48988=CARTESIAN_POINT('Origin',(-10.7196129999499,-1.5,120.038479161527));
#48989=CARTESIAN_POINT('',(-10.7196129999499,-1.5,120.038479161527));
#48990=CARTESIAN_POINT('',(-10.2010167633031,-1.5,120.752265645672));
#48991=CARTESIAN_POINT('',(-10.7196129999499,-1.45,120.038479161527));
#48992=CARTESIAN_POINT('',(-10.7196129999499,-1.5,120.038479161527));
#48993=CARTESIAN_POINT('',(-10.7196129999499,-1.45,120.038479161527));
#48994=CARTESIAN_POINT('Origin',(-10.4364570519187,-1.5,119.832754323225));
#48995=CARTESIAN_POINT('',(-10.4364570519187,-1.5,119.832754323225));
#48996=CARTESIAN_POINT('',(-8.53682476260632,-1.5,118.452590677467));
#48997=CARTESIAN_POINT('',(-10.4364570519187,-1.45,119.832754323225));
#48998=CARTESIAN_POINT('',(-10.4364570519187,-1.5,119.832754323225));
#48999=CARTESIAN_POINT('',(-10.4364570519187,-1.45,119.832754323225));
#49000=CARTESIAN_POINT('Origin',(-10.3659228216436,-1.5,119.92983636255));
#49001=CARTESIAN_POINT('',(-9.88259370013425,-1.5,120.595081827033));
#49002=CARTESIAN_POINT('',(-10.3659228216436,-1.45,119.92983636255));
#49003=CARTESIAN_POINT('Origin',(-10.5427679107967,-1.45,119.984157762038));
#49004=CARTESIAN_POINT('Origin',(-8.44,-1.5,121.2));
#49005=CARTESIAN_POINT('',(-8.44,-1.5,121.2));
#49006=CARTESIAN_POINT('',(-8.44,-1.5,120.85));
#49007=CARTESIAN_POINT('',(-8.44,-1.5,119.85));
#49008=CARTESIAN_POINT('',(-8.44,-1.45,121.2));
#49009=CARTESIAN_POINT('',(-8.44,-1.5,121.2));
#49010=CARTESIAN_POINT('',(-8.44,-1.45,120.85));
#49011=CARTESIAN_POINT('',(-8.44,-1.45,121.2));
#49012=CARTESIAN_POINT('',(-8.44,-1.5,120.85));
#49013=CARTESIAN_POINT('Origin',(-8.56,-1.5,121.2));
#49014=CARTESIAN_POINT('',(-8.56,-1.5,121.2));
#49015=CARTESIAN_POINT('',(-7.08,-1.5,121.2));
#49016=CARTESIAN_POINT('',(-8.56,-1.45,121.2));
#49017=CARTESIAN_POINT('',(-8.56,-1.5,121.2));
#49018=CARTESIAN_POINT('',(-8.56,-1.45,121.2));
#49019=CARTESIAN_POINT('Origin',(-8.56,-1.5,120.85));
#49020=CARTESIAN_POINT('',(-8.56,-1.5,120.85));
#49021=CARTESIAN_POINT('',(-8.56,-1.5,119.675));
#49022=CARTESIAN_POINT('',(-8.56,-1.45,120.85));
#49023=CARTESIAN_POINT('',(-8.56,-1.5,120.85));
#49024=CARTESIAN_POINT('',(-8.56,-1.45,120.85));
#49025=CARTESIAN_POINT('Origin',(-8.44,-1.5,120.85));
#49026=CARTESIAN_POINT('',(-7.02,-1.5,120.85));
#49027=CARTESIAN_POINT('',(-8.44,-1.45,120.85));
#49028=CARTESIAN_POINT('Origin',(-8.5,-1.45,121.025));
#49029=CARTESIAN_POINT('Origin',(-7.22076525925192,-1.5,120.878478185324));
#49030=CARTESIAN_POINT('',(-7.22076525925192,-1.5,120.878478185324));
#49031=CARTESIAN_POINT('',(-7.49315955909565,-1.5,120.343874270811));
#49032=CARTESIAN_POINT('',(-7.53479674181235,-1.5,120.262156698592));
#49033=CARTESIAN_POINT('',(-7.22076525925192,-1.45,120.878478185324));
#49034=CARTESIAN_POINT('',(-7.22076525925192,-1.5,120.878478185324));
#49035=CARTESIAN_POINT('',(-7.49315955909565,-1.45,120.343874270811));
#49036=CARTESIAN_POINT('',(-7.22076525925192,-1.45,120.878478185324));
#49037=CARTESIAN_POINT('',(-7.49315955909565,-1.5,120.343874270811));
#49038=CARTESIAN_POINT('Origin',(-7.32768604215453,-1.5,120.932957045293));
#49039=CARTESIAN_POINT('',(-7.32768604215453,-1.5,120.932957045293));
#49040=CARTESIAN_POINT('',(-6.14981153851683,-1.5,120.332800009379));
#49041=CARTESIAN_POINT('',(-7.32768604215453,-1.45,120.932957045293));
#49042=CARTESIAN_POINT('',(-7.32768604215453,-1.5,120.932957045293));
#49043=CARTESIAN_POINT('',(-7.32768604215453,-1.45,120.932957045293));
#49044=CARTESIAN_POINT('Origin',(-7.60008034199825,-1.5,120.39835313078));
#49045=CARTESIAN_POINT('',(-7.60008034199825,-1.5,120.39835313078));
#49046=CARTESIAN_POINT('',(-7.77791467463682,-1.5,120.049333601304));
#49047=CARTESIAN_POINT('',(-7.60008034199825,-1.45,120.39835313078));
#49048=CARTESIAN_POINT('',(-7.60008034199825,-1.5,120.39835313078));
#49049=CARTESIAN_POINT('',(-7.60008034199825,-1.45,120.39835313078));
#49050=CARTESIAN_POINT('Origin',(-7.49315955909565,-1.5,120.343874270811));
#49051=CARTESIAN_POINT('',(-6.36874544690924,-1.5,119.770956664882));
#49052=CARTESIAN_POINT('',(-7.49315955909565,-1.45,120.343874270811));
#49053=CARTESIAN_POINT('Origin',(-7.41042280062509,-1.45,120.638415658052));
#49054=CARTESIAN_POINT('Origin',(-5.82385541249071,-1.5,118.863111755173));
#49055=CARTESIAN_POINT('',(-5.82385541249071,-1.5,118.863111755173));
#49056=CARTESIAN_POINT('',(-6.4164684168478,-1.5,118.769251076149));
#49057=CARTESIAN_POINT('',(-5.74271869798015,-1.5,118.87596254829));
#49058=CARTESIAN_POINT('',(-5.82385541249071,-1.45,118.863111755173));
#49059=CARTESIAN_POINT('',(-5.82385541249071,-1.5,118.863111755173));
#49060=CARTESIAN_POINT('',(-6.4164684168478,-1.45,118.769251076149));
#49061=CARTESIAN_POINT('',(-5.82385541249071,-1.45,118.863111755173));
#49062=CARTESIAN_POINT('',(-6.4164684168478,-1.5,118.769251076149));
#49063=CARTESIAN_POINT('Origin',(-5.84262754829554,-1.5,118.981634356044));
#49064=CARTESIAN_POINT('',(-5.84262754829554,-1.5,118.981634356044));
#49065=CARTESIAN_POINT('',(-5.80245048865833,-1.5,118.727966384905));
#49066=CARTESIAN_POINT('',(-5.84262754829554,-1.45,118.981634356044));
#49067=CARTESIAN_POINT('',(-5.84262754829554,-1.5,118.981634356044));
#49068=CARTESIAN_POINT('',(-5.84262754829554,-1.45,118.981634356044));
#49069=CARTESIAN_POINT('Origin',(-6.43524055265262,-1.5,118.88777367702));
#49070=CARTESIAN_POINT('',(-6.43524055265262,-1.5,118.88777367702));
#49071=CARTESIAN_POINT('',(-6.05779733596353,-1.5,118.94755480965));
#49072=CARTESIAN_POINT('',(-6.43524055265262,-1.45,118.88777367702));
#49073=CARTESIAN_POINT('',(-6.43524055265262,-1.5,118.88777367702));
#49074=CARTESIAN_POINT('',(-6.43524055265262,-1.45,118.88777367702));
#49075=CARTESIAN_POINT('Origin',(-6.4164684168478,-1.5,118.769251076149));
#49076=CARTESIAN_POINT('',(-6.385677425113,-1.5,118.574844405445));
#49077=CARTESIAN_POINT('',(-6.4164684168478,-1.45,118.769251076149));
#49078=CARTESIAN_POINT('Origin',(-6.12954798257167,-1.45,118.875442716097));
#49079=CARTESIAN_POINT('Origin',(-6.63323809766752,-1.5,116.548385283925));
#49080=CARTESIAN_POINT('',(-6.63323809766752,-1.5,116.548385283925));
#49081=CARTESIAN_POINT('',(-7.05750216637944,-1.5,116.972649352637));
#49082=CARTESIAN_POINT('',(-6.86283225226936,-1.5,116.777979438527));
#49083=CARTESIAN_POINT('',(-6.63323809766752,-1.45,116.548385283925));
#49084=CARTESIAN_POINT('',(-6.63323809766752,-1.5,116.548385283925));
#49085=CARTESIAN_POINT('',(-7.05750216637944,-1.45,116.972649352637));
#49086=CARTESIAN_POINT('',(-6.63323809766752,-1.45,116.548385283925));
#49087=CARTESIAN_POINT('',(-7.05750216637944,-1.5,116.972649352637));
#49088=CARTESIAN_POINT('Origin',(-6.54838528392513,-1.5,116.633238097668));
#49089=CARTESIAN_POINT('',(-6.54838528392513,-1.5,116.633238097668));
#49090=CARTESIAN_POINT('',(-5.84459848736068,-1.5,117.337024894232));
#49091=CARTESIAN_POINT('',(-6.54838528392513,-1.45,116.633238097668));
#49092=CARTESIAN_POINT('',(-6.54838528392513,-1.5,116.633238097668));
#49093=CARTESIAN_POINT('',(-6.54838528392513,-1.45,116.633238097668));
#49094=CARTESIAN_POINT('Origin',(-6.97264935263706,-1.5,117.057502166379));
#49095=CARTESIAN_POINT('',(-6.97264935263706,-1.5,117.057502166379));
#49096=CARTESIAN_POINT('',(-6.99011147288294,-1.5,117.074964286625));
#49097=CARTESIAN_POINT('',(-6.97264935263706,-1.45,117.057502166379));
#49098=CARTESIAN_POINT('',(-6.97264935263706,-1.5,117.057502166379));
#49099=CARTESIAN_POINT('',(-6.97264935263706,-1.45,117.057502166379));
#49100=CARTESIAN_POINT('Origin',(-7.05750216637944,-1.5,116.972649352637));
#49101=CARTESIAN_POINT('',(-6.31128896294379,-1.5,117.718862556073));
#49102=CARTESIAN_POINT('',(-7.05750216637944,-1.45,116.972649352637));
#49103=CARTESIAN_POINT('Origin',(-6.80294372515229,-1.45,116.802943725152));
#49104=CARTESIAN_POINT('Origin',(-5.6,-1.5,118.5));
#49105=CARTESIAN_POINT('',(-11.4,-1.5,118.5));
#49106=CARTESIAN_POINT('Origin',(-8.5,-1.5,118.5));
#49107=CARTESIAN_POINT('Origin',(-8.5,-1.625,118.5));
#49108=CARTESIAN_POINT('',(-11.4,-1.7,118.5));
#49109=CARTESIAN_POINT('',(-11.4,-1.625,118.5));
#49110=CARTESIAN_POINT('Origin',(-8.5,-1.7,118.5));
#49111=CARTESIAN_POINT('Origin',(-5.55,1.4,118.5));
#49112=CARTESIAN_POINT('',(-11.45,1.4,118.5));
#49113=CARTESIAN_POINT('Origin',(-8.5,1.4,118.5));
#49114=CARTESIAN_POINT('Origin',(-8.5,1.3,118.5));
#49115=CARTESIAN_POINT('',(-11.65,1.2,118.5));
#49116=CARTESIAN_POINT('Origin',(-8.5,1.2,118.5));
#49117=CARTESIAN_POINT('',(-11.55,1.3,118.5));
#49118=CARTESIAN_POINT('Origin',(-8.5,0.,118.5));
#49119=CARTESIAN_POINT('',(-11.65,-1.2,118.5));
#49120=CARTESIAN_POINT('Origin',(-8.5,-1.2,118.5));
#49121=CARTESIAN_POINT('',(-11.65,0.,118.5));
#49122=CARTESIAN_POINT('Origin',(-5.2,-1.2,118.5));
#49123=CARTESIAN_POINT('',(-11.8,-1.2,118.5));
#49124=CARTESIAN_POINT('Origin',(-8.5,-1.2,118.5));
#49125=CARTESIAN_POINT('Origin',(-8.5,-1.4,118.5));
#49126=CARTESIAN_POINT('',(-11.8,-1.6,118.5));
#49127=CARTESIAN_POINT('Origin',(-8.5,-1.6,118.5));
#49128=CARTESIAN_POINT('',(-11.8,-1.4,118.5));
#49129=CARTESIAN_POINT('Origin',(-8.5,-1.65,118.5));
#49130=CARTESIAN_POINT('',(-11.7,-1.7,118.5));
#49131=CARTESIAN_POINT('Origin',(-8.5,-1.7,118.5));
#49132=CARTESIAN_POINT('',(-11.75,-1.65,118.5));
#49133=CARTESIAN_POINT('Origin',(-8.5,-1.7,118.5));
#71459=UNCERTAINTY_MEASURE_WITH_UNIT(LENGTH_MEASURE(0.001),#71493,
'DISTANCE_ACCURACY_VALUE',
'Maximum model space distance between geometric entities at asserted c
onnectivities');
#71471=UNCERTAINTY_MEASURE_WITH_UNIT(LENGTH_MEASURE(0.001),#71493,
'DISTANCE_ACCURACY_VALUE',
'Maximum model space distance between geometric entities at asserted c
onnectivities');
#71480=(
GEOMETRIC_REPRESENTATION_CONTEXT(3)
GLOBAL_UNCERTAINTY_ASSIGNED_CONTEXT((#71459))
GLOBAL_UNIT_ASSIGNED_CONTEXT((#71493,#71495,#71496))
REPRESENTATION_CONTEXT('','3D')
);
#71492=(
GEOMETRIC_REPRESENTATION_CONTEXT(3)
GLOBAL_UNCERTAINTY_ASSIGNED_CONTEXT((#71471))
GLOBAL_UNIT_ASSIGNED_CONTEXT((#71493,#71495,#71496))
REPRESENTATION_CONTEXT('','3D')
);
#71493=(
LENGTH_UNIT()
NAMED_UNIT(*)
SI_UNIT(.CENTI.,.METRE.)
);
#71495=(
NAMED_UNIT(*)
PLANE_ANGLE_UNIT()
SI_UNIT($,.RADIAN.)
);
#71496=(
NAMED_UNIT(*)
SI_UNIT($,.STERADIAN.)
SOLID_ANGLE_UNIT()
);
#71505=SHAPE_DEFINITION_REPRESENTATION(#71525,#71610);
#71525=PRODUCT_DEFINITION_SHAPE('',$,#71631);
#71610=SHAPE_REPRESENTATION('',(#29878),#71480);
#71622=PRODUCT_DEFINITION_CONTEXT('part definition',#71684,'design');
#71631=PRODUCT_DEFINITION('2026-10-19-03-22-43-799',
'13_Pressure_Gauge_D63_0-20T',#71651,#71622);
#71651=PRODUCT_DEFINITION_FORMATION('',$,#71694);
#71684=APPLICATION_CONTEXT(
'Core Data for Automotive Mechanical Design Process');
#71685=PRODUCT_CONTEXT('part definition',#71684,'mechanical');
#71694=PRODUCT('2026-10-19-03-22-43-799','13_Pressure_Gauge_D63_0-20T',
$,(#71685));
#71895=COLOUR_RGB('Off White',0.89,0.88,0.83);
#71896=FILL_AREA_STYLE_COLOUR('',#71895);
#71897=FILL_AREA_STYLE('',(#71896));
#71898=SURFACE_STYLE_FILL_AREA(#71897);
#71899=SURFACE_SIDE_STYLE('',(#71898));
#71900=SURFACE_STYLE_USAGE(.BOTH.,#71899);
#71901=PRESENTATION_STYLE_ASSIGNMENT((#71900));
ENDSEC;
END-ISO-10303-21;
